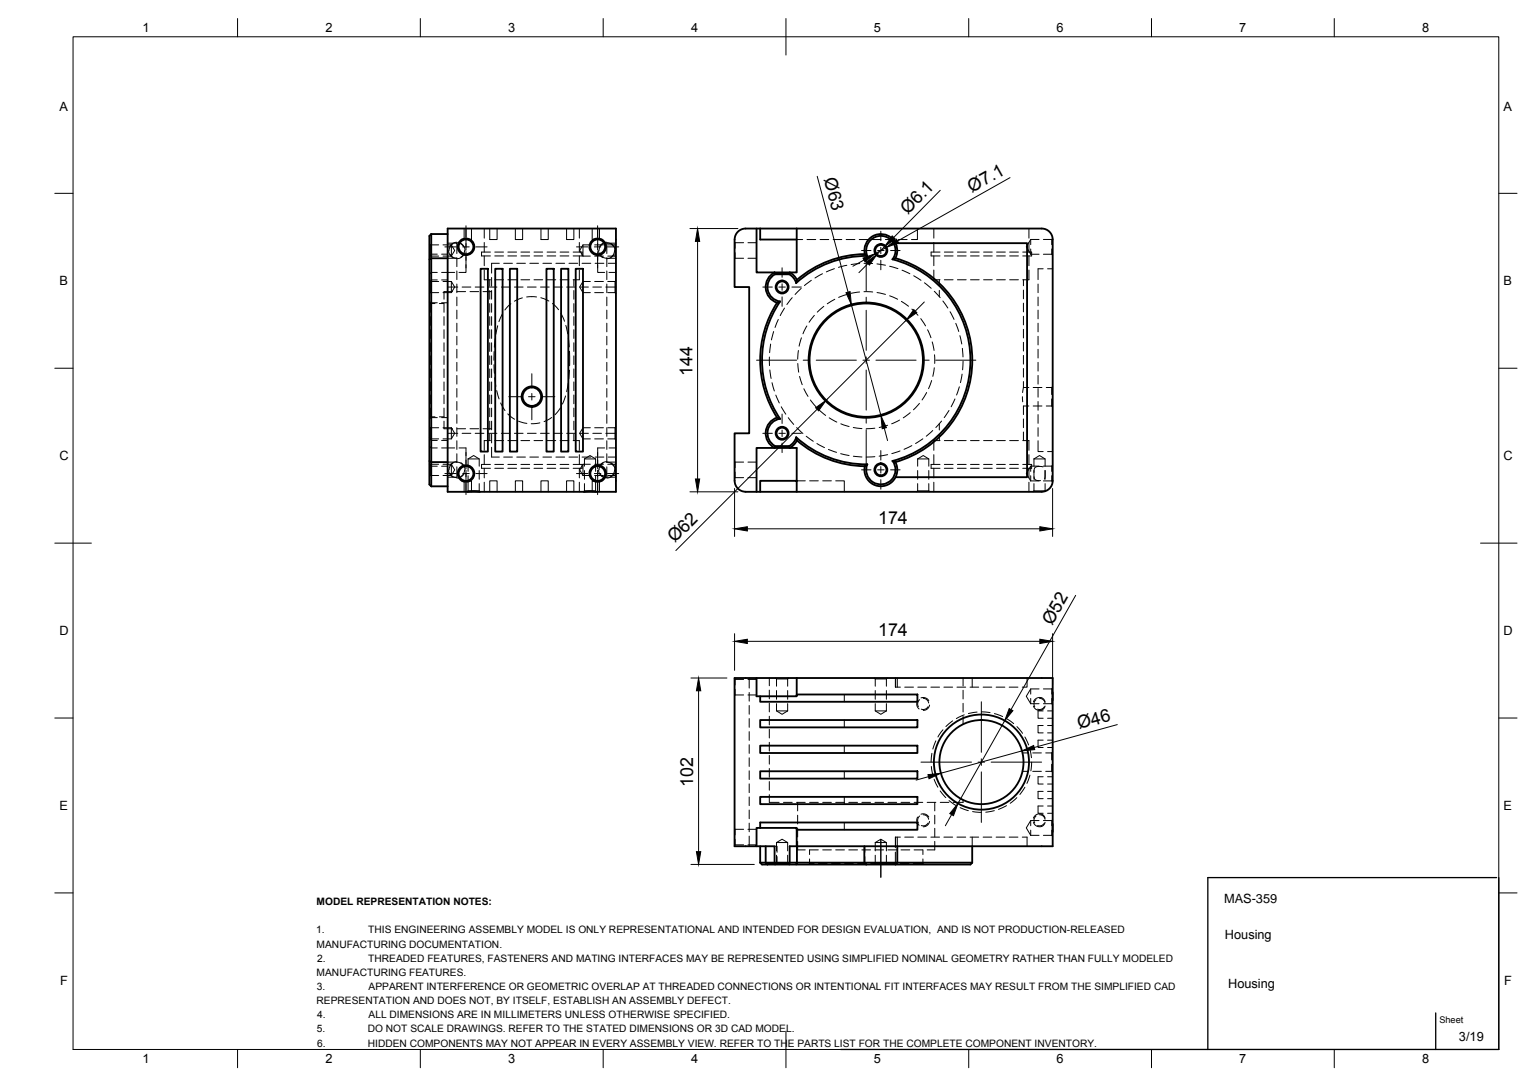
ISO-10303-21;
HEADER;
/* Generated by software containing ST-Developer
 * from STEP Tools, Inc. (www.steptools.com) 
 */

FILE_DESCRIPTION(
/* description */ (''),
/* implementation_level */ '2;1');

FILE_NAME(
/* name */ 'Housing.step',
/* time_stamp */ '2026-10-15T14:25:16-07:00',
/* author */ (''),
/* organization */ (''),
/* preprocessor_version */ 'ST-DEVELOPER v20.2',
/* originating_system */ 'Autodesk Translation Framework v15.15.0.0',
/* authorisation */ '');

FILE_SCHEMA (('AUTOMOTIVE_DESIGN { 1 0 10303 214 3 1 1 }'));
ENDSEC;

DATA;
#10=MECHANICAL_DESIGN_GEOMETRIC_PRESENTATION_REPRESENTATION('',(#323),#86429);
#287=SHAPE_REPRESENTATION_RELATIONSHIP('SRR','None',#86502,#305);
#305=ADVANCED_BREP_SHAPE_REPRESENTATION('',(#341),#86411);
#323=STYLED_ITEM('',(#86601),#341);
#341=MANIFOLD_SOLID_BREP('Body1',#15613);
#359=ELLIPSE('',#15940,151.19389506818,3.23363209990621);
#360=ELLIPSE('',#15943,151.194075359537,3.2336340714008);
#361=ELLIPSE('',#15952,151.194380471967,3.23363740533001);
#362=ELLIPSE('',#15955,151.194647853758,3.23364033017112);
#363=B_SPLINE_CURVE_WITH_KNOTS('',3,(#21563,#21564,#21565,#21566),
 .UNSPECIFIED.,.F.,.F.,(4,4),(-0.201492965018242,0.),.UNSPECIFIED.);
#364=B_SPLINE_CURVE_WITH_KNOTS('',3,(#21569,#21570,#21571,#21572),
 .UNSPECIFIED.,.F.,.F.,(4,4),(-0.195594022319034,0.),.UNSPECIFIED.);
#365=B_SPLINE_CURVE_WITH_KNOTS('',3,(#21589,#21590,#21591,#21592),
 .UNSPECIFIED.,.F.,.F.,(4,4),(-0.201492965018205,0.),.UNSPECIFIED.);
#366=B_SPLINE_CURVE_WITH_KNOTS('',3,(#21598,#21599,#21600,#21601),
 .UNSPECIFIED.,.F.,.F.,(4,4),(-0.201492965018185,0.),.UNSPECIFIED.);
#367=B_SPLINE_CURVE_WITH_KNOTS('',3,(#21620,#21621,#21622,#21623),
 .UNSPECIFIED.,.F.,.F.,(4,4),(-0.201492965018191,0.),.UNSPECIFIED.);
#368=B_SPLINE_CURVE_WITH_KNOTS('',3,(#21629,#21630,#21631,#21632),
 .UNSPECIFIED.,.F.,.F.,(4,4),(-0.195594022319061,0.),.UNSPECIFIED.);
#369=B_SPLINE_CURVE_WITH_KNOTS('',3,(#21638,#21639,#21640,#21641),
 .UNSPECIFIED.,.F.,.F.,(4,4),(-0.195594022319045,0.),.UNSPECIFIED.);
#370=B_SPLINE_CURVE_WITH_KNOTS('',3,(#21647,#21648,#21649,#21650),
 .UNSPECIFIED.,.F.,.F.,(4,4),(-0.195594022319043,0.),.UNSPECIFIED.);
#371=B_SPLINE_CURVE_WITH_KNOTS('',3,(#21681,#21682,#21683,#21684,#21685,
#21686,#21687,#21688,#21689,#21690),.UNSPECIFIED.,.F.,.F.,(4,2,2,2,4),(-3.05436467918173,
-2.86345905577985,-2.67255343237797,-2.48166347088213,-2.2907735093863),
 .UNSPECIFIED.);
#372=B_SPLINE_CURVE_WITH_KNOTS('',3,(#21691,#21692,#21693,#21694,#21695,
#21696,#21697,#21698,#21699,#21700,#21701,#21702,#21703,#21704,#21705,#21706,
#21707,#21708,#21709,#21710,#21711,#21712,#21713,#21714,#21715,#21716),
 .UNSPECIFIED.,.F.,.F.,(4,2,2,2,2,2,2,2,2,2,2,2,4),(-2.2907735093863,-2.09988354789047,
-1.90899358639463,-1.71808796299275,-1.52718233959087,-1.33627671618898,
-1.1453710927871,-0.954481131291268,-0.763591169795433,-0.572701208299599,
-0.381811246803764,-0.190905623401882,0.),.UNSPECIFIED.);
#373=B_SPLINE_CURVE_WITH_KNOTS('',3,(#21733,#21734,#21735,#21736,#21737,
#21738,#21739,#21740,#21741,#21742,#21743,#21744,#21745,#21746),
 .UNSPECIFIED.,.F.,.F.,(4,2,2,2,2,2,4),(-1.32169585665546,-1.18688181797703,
-1.0520677792986,-0.988183485413416,-0.924299191528231,-0.792573559927981,
-0.660847928327731),.UNSPECIFIED.);
#374=B_SPLINE_CURVE_WITH_KNOTS('',3,(#21748,#21749,#21750,#21751,#21752,
#21753,#21754,#21755,#21756,#21757,#21758,#21759,#21760,#21761),
 .UNSPECIFIED.,.F.,.F.,(4,2,2,2,2,2,4),(0.660847928327731,0.792573559927981,
0.924299191528231,0.988183485413416,1.0520677792986,1.18688181797703,1.32169585665546),
 .UNSPECIFIED.);
#375=B_SPLINE_CURVE_WITH_KNOTS('',3,(#21765,#21766,#21767,#21768,#21769,
#21770,#21771,#21772,#21773,#21774,#21775,#21776,#21777,#21778,#21779,#21780,
#21781,#21782,#21783,#21784,#21785,#21786,#21787,#21788,#21789,#21790,#21791),
 .UNSPECIFIED.,.F.,.F.,(4,2,2,2,2,2,3,2,2,2,2,2,4),(-0.660847928327731,
-0.529122296727481,-0.39739666512723,-0.333512371242046,-0.269628077356861,
-0.134814038678431,0.,0.13481403867843,0.269628077356861,0.333512371242045,
0.39739666512723,0.52912229672748,0.660847928327731),.UNSPECIFIED.);
#376=B_SPLINE_CURVE_WITH_KNOTS('',3,(#21798,#21799,#21800,#21801,#21802,
#21803,#21804,#21805,#21806,#21807),.UNSPECIFIED.,.F.,.F.,(4,2,2,2,4),(0.858794530961258,
0.902694826940309,1.07577532936191,1.25459835745813,1.29336839957273),
 .UNSPECIFIED.);
#377=B_SPLINE_CURVE_WITH_KNOTS('',3,(#21893,#21894,#21895,#21896,#21897,
#21898,#21899,#21900,#21901,#21902,#21903,#21904,#21905,#21906,#21907,#21908,
#21909,#21910,#21911,#21912,#21913,#21914,#21915,#21916,#21917,#21918),
 .UNSPECIFIED.,.F.,.F.,(4,2,2,2,2,2,2,2,2,2,2,2,4),(-1.32169585665546,-1.18688181797703,
-1.0520677792986,-0.988183485413416,-0.924299191528231,-0.792573559927981,
-0.660847928327731,-0.529122296727481,-0.39739666512723,-0.333512371242046,
-0.269628077356861,-0.134814038678431,0.),.UNSPECIFIED.);
#378=B_SPLINE_CURVE_WITH_KNOTS('',3,(#21919,#21920,#21921,#21922,#21923,
#21924,#21925,#21926,#21927,#21928,#21929,#21930,#21931,#21932,#21933,#21934,
#21935,#21936,#21937,#21938,#21939,#21940,#21941,#21942,#21943,#21944),
 .UNSPECIFIED.,.F.,.F.,(4,2,2,2,2,2,2,2,2,2,2,2,4),(0.,0.13481403867843,
0.269628077356861,0.333512371242045,0.39739666512723,0.52912229672748,0.660847928327731,
0.792573559927981,0.924299191528231,0.988183485413416,1.0520677792986,1.18688181797703,
1.32169585665546),.UNSPECIFIED.);
#379=B_SPLINE_CURVE_WITH_KNOTS('',3,(#21947,#21948,#21949,#21950,#21951,
#21952,#21953,#21954,#21955,#21956),.UNSPECIFIED.,.F.,.F.,(4,2,2,2,4),(0.877716942395265,
0.916486984509874,1.09531001260609,1.26839051502769,1.31229081100675),
 .UNSPECIFIED.);
#380=B_SPLINE_CURVE_WITH_KNOTS('',3,(#21958,#21959,#21960,#21961,#21962,
#21963,#21964,#21965,#21966,#21967,#21968,#21969,#21970,#21971,#21972,#21973,
#21974,#21975,#21976,#21977,#21978,#21979,#21980),.UNSPECIFIED.,.F.,.F.,
(4,2,2,2,2,3,2,2,2,2,4),(1.51638402057123,1.52276019461865,1.58643945940805,
1.65011872419746,1.7823849294906,1.91465113478373,2.04691734007687,2.17918354537001,
2.24286281015941,2.30654207494882,2.31291824899624),.UNSPECIFIED.);
#381=B_SPLINE_CURVE_WITH_KNOTS('',3,(#21981,#21982,#21983,#21984,#21985,
#21986,#21987,#21988,#21989,#21990,#21991,#21992,#21993,#21994,#21995,#21996,
#21997,#21998,#21999,#22000,#22001,#22002,#22003),.UNSPECIFIED.,.F.,.F.,
(4,2,2,2,2,3,2,2,2,2,4),(1.51638402057122,1.52276019461865,1.58643945940805,
1.65011872419746,1.7823849294906,1.91465113478373,2.04691734007687,2.17918354537001,
2.24286281015942,2.30654207494882,2.31291824899624),.UNSPECIFIED.);
#382=B_SPLINE_CURVE_WITH_KNOTS('',3,(#22016,#22017,#22018,#22019,#22020,
#22021,#22022,#22023,#22024,#22025),.UNSPECIFIED.,.F.,.F.,(4,2,2,2,4),(0.877716942395273,
0.916486984509874,1.09531001260609,1.26839051502769,1.31229081100674),
 .UNSPECIFIED.);
#383=B_SPLINE_CURVE_WITH_KNOTS('',3,(#22028,#22029,#22030,#22031,#22032,
#22033,#22034,#22035,#22036,#22037),.UNSPECIFIED.,.F.,.F.,(4,2,2,2,4),(0.858794530961249,
0.902694826940311,1.07577532936191,1.25459835745813,1.29336839957274),
 .UNSPECIFIED.);
#384=B_SPLINE_CURVE_WITH_KNOTS('',3,(#22453,#22454,#22455,#22456,#22457,
#22458,#22459,#22460,#22461,#22462,#22463,#22464,#22465,#22466,#22467,#22468,
#22469,#22470),.UNSPECIFIED.,.F.,.F.,(4,2,2,2,2,2,2,2,4),(-9.41073061373359,
-8.52189532994956,-7.63306004616553,-6.7442247623815,-5.85538947859747,
-5.5678834356648,-5.28037739273213,-4.99287134979946,-4.70536530686679),
 .UNSPECIFIED.);
#385=B_SPLINE_CURVE_WITH_KNOTS('',3,(#22472,#22473,#22474,#22475,#22476,
#22477,#22478,#22479,#22480,#22481,#22482,#22483,#22484,#22485,#22486,#22487,
#22488,#22489),.UNSPECIFIED.,.F.,.F.,(4,2,2,2,2,2,2,2,4),(4.70536530686679,
4.99287134979946,5.28037739273213,5.5678834356648,5.85538947859747,6.7442247623815,
7.63306004616553,8.52189532994956,9.41073061373359),.UNSPECIFIED.);
#386=B_SPLINE_CURVE_WITH_KNOTS('',3,(#22493,#22494,#22495,#22496,#22497,
#22498,#22499,#22500,#22501,#22502,#22503,#22504,#22505,#22506,#22507,#22508,
#22509,#22510,#22511,#22512,#22513,#22514,#22515,#22516,#22517,#22518,#22519,
#22520,#22521,#22522,#22523,#22524,#22525,#22526,#22527),.UNSPECIFIED.,
 .F.,.F.,(4,2,2,2,2,2,2,2,3,2,2,2,2,2,2,2,4),(-4.70536530686679,-4.41785926393413,
-4.13035322100146,-3.84284717806879,-3.55534113513612,-2.66650585135209,
-1.77767056756806,-0.888835283784031,0.,0.888835283784029,1.77767056756806,
2.66650585135209,3.55534113513612,3.84284717806879,4.13035322100146,4.41785926393413,
4.70536530686679),.UNSPECIFIED.);
#1145=CONICAL_SURFACE('',#15935,5.75,0.785398163397448);
#1146=CONICAL_SURFACE('',#15938,0.85,0.78539816339745);
#1147=CONICAL_SURFACE('',#15944,0.85,0.78539816339745);
#1148=CONICAL_SURFACE('',#15947,5.75,0.785398163397453);
#1149=CONICAL_SURFACE('',#15950,0.85,0.78539816339745);
#1150=CONICAL_SURFACE('',#15956,0.85,0.78539816339745);
#1151=CONICAL_SURFACE('',#15959,5.75,0.785398163397448);
#1152=CONICAL_SURFACE('',#15962,0.85,0.785398163397452);
#1153=CONICAL_SURFACE('',#15965,5.75,0.785398163397448);
#1154=CONICAL_SURFACE('',#15968,0.85,0.785398163397452);
#1155=CONICAL_SURFACE('',#15985,0.5575,0.785398163397445);
#1156=CONICAL_SURFACE('',#15987,0.2025,1.02974425867666);
#1157=CONICAL_SURFACE('',#15991,0.455,0.785398163397457);
#1158=CONICAL_SURFACE('',#16001,0.2025,1.02974425867666);
#1159=CONICAL_SURFACE('',#16005,0.455000000000001,0.785398163397459);
#1160=CONICAL_SURFACE('',#16008,0.2025,1.02974425867666);
#1161=CONICAL_SURFACE('',#16012,0.455,0.785398163397457);
#1162=CONICAL_SURFACE('',#16015,0.2025,1.02974425867666);
#1163=CONICAL_SURFACE('',#16019,0.455000000000001,0.785398163397459);
#1164=CONICAL_SURFACE('',#16020,0.1525,1.02974425867665);
#1165=CONICAL_SURFACE('',#16024,0.355,0.785398163397444);
#1166=CONICAL_SURFACE('',#16025,0.1525,1.02974425867665);
#1167=CONICAL_SURFACE('',#16029,0.355,0.785398163397446);
#1168=CONICAL_SURFACE('',#16031,0.1525,1.02974425867665);
#1169=CONICAL_SURFACE('',#16035,0.355,0.785398163397446);
#1170=CONICAL_SURFACE('',#16036,0.1525,1.02974425867665);
#1171=CONICAL_SURFACE('',#16040,0.355,0.785398163397444);
#1172=CONICAL_SURFACE('',#16042,0.1525,1.02974425867665);
#1173=CONICAL_SURFACE('',#16046,0.355,0.785398163397444);
#1174=CONICAL_SURFACE('',#16047,0.1525,1.02974425867665);
#1175=CONICAL_SURFACE('',#16051,0.355,0.785398163397444);
#1176=CONICAL_SURFACE('',#16053,0.1525,1.02974425867665);
#1177=CONICAL_SURFACE('',#16057,0.355,0.785398163397444);
#1178=CONICAL_SURFACE('',#16058,0.1525,1.02974425867665);
#1179=CONICAL_SURFACE('',#16062,0.355,0.785398163397444);
#1180=CONICAL_SURFACE('',#16064,0.1525,1.02974425867665);
#1181=CONICAL_SURFACE('',#16068,0.355,0.785398163397451);
#1182=CONICAL_SURFACE('',#16069,0.1525,1.02974425867665);
#1183=CONICAL_SURFACE('',#16073,0.355,0.785398163397448);
#1184=CONICAL_SURFACE('',#16074,0.1525,1.02974425867665);
#1185=CONICAL_SURFACE('',#16078,0.355,0.785398163397451);
#1186=CONICAL_SURFACE('',#16079,0.1525,1.02974425867665);
#1187=CONICAL_SURFACE('',#16083,0.355,0.785398163397448);
#1188=CONICAL_SURFACE('',#16087,0.462499999999999,0.785398163397447);
#1189=CONICAL_SURFACE('',#16092,0.4625,0.785398163397444);
#1190=CONICAL_SURFACE('',#16097,0.462499999999999,0.785398163397447);
#1191=CONICAL_SURFACE('',#16102,0.4625,0.785398163397444);
#1192=CONICAL_SURFACE('',#16199,3.155,0.785398163397444);
#1351=CYLINDRICAL_SURFACE('',#15906,5.8);
#1352=CYLINDRICAL_SURFACE('',#15909,0.9);
#1353=CYLINDRICAL_SURFACE('',#15915,0.9);
#1354=CYLINDRICAL_SURFACE('',#15971,0.9);
#1355=CYLINDRICAL_SURFACE('',#15972,5.8);
#1356=CYLINDRICAL_SURFACE('',#15973,0.9);
#1357=CYLINDRICAL_SURFACE('',#15974,5.8);
#1358=CYLINDRICAL_SURFACE('',#15975,0.9);
#1359=CYLINDRICAL_SURFACE('',#15976,5.8);
#1360=CYLINDRICAL_SURFACE('',#15983,0.505);
#1361=CYLINDRICAL_SURFACE('',#15989,0.405);
#1362=CYLINDRICAL_SURFACE('',#16003,0.405);
#1363=CYLINDRICAL_SURFACE('',#16006,0.6);
#1364=CYLINDRICAL_SURFACE('',#16010,0.405);
#1365=CYLINDRICAL_SURFACE('',#16013,0.6);
#1366=CYLINDRICAL_SURFACE('',#16017,0.405);
#1367=CYLINDRICAL_SURFACE('',#16022,0.305);
#1368=CYLINDRICAL_SURFACE('',#16027,0.305);
#1369=CYLINDRICAL_SURFACE('',#16033,0.305);
#1370=CYLINDRICAL_SURFACE('',#16038,0.305);
#1371=CYLINDRICAL_SURFACE('',#16044,0.305);
#1372=CYLINDRICAL_SURFACE('',#16049,0.305);
#1373=CYLINDRICAL_SURFACE('',#16055,0.305);
#1374=CYLINDRICAL_SURFACE('',#16060,0.305);
#1375=CYLINDRICAL_SURFACE('',#16066,0.305);
#1376=CYLINDRICAL_SURFACE('',#16071,0.305);
#1377=CYLINDRICAL_SURFACE('',#16076,0.305);
#1378=CYLINDRICAL_SURFACE('',#16081,0.305);
#1379=CYLINDRICAL_SURFACE('',#16084,0.425);
#1380=CYLINDRICAL_SURFACE('',#16089,0.425000000000001);
#1381=CYLINDRICAL_SURFACE('',#16094,0.425);
#1382=CYLINDRICAL_SURFACE('',#16099,0.425000000000001);
#1383=CYLINDRICAL_SURFACE('',#16120,0.9);
#1384=CYLINDRICAL_SURFACE('',#16122,0.9);
#1385=CYLINDRICAL_SURFACE('',#16123,0.9);
#1386=CYLINDRICAL_SURFACE('',#16164,2.6);
#1387=CYLINDRICAL_SURFACE('',#16168,2.75);
#1388=CYLINDRICAL_SURFACE('',#16172,2.6);
#1389=CYLINDRICAL_SURFACE('',#16176,2.3);
#1390=CYLINDRICAL_SURFACE('',#16180,2.6);
#1391=CYLINDRICAL_SURFACE('',#16184,2.75);
#1392=CYLINDRICAL_SURFACE('',#16188,2.6);
#1393=CYLINDRICAL_SURFACE('',#16189,5.3);
#1394=CYLINDRICAL_SURFACE('',#16193,3.75);
#1395=CYLINDRICAL_SURFACE('',#16197,3.1);
#1396=CYLINDRICAL_SURFACE('',#16200,5.8);
#1397=CYLINDRICAL_SURFACE('',#16201,0.6);
#1398=CYLINDRICAL_SURFACE('',#16202,0.6);
#1602=FACE_BOUND('',#3290,.T.);
#1603=FACE_BOUND('',#3291,.T.);
#1604=FACE_BOUND('',#3292,.T.);
#1605=FACE_BOUND('',#3293,.T.);
#1606=FACE_BOUND('',#3294,.T.);
#1607=FACE_BOUND('',#3328,.T.);
#1608=FACE_BOUND('',#3329,.T.);
#1609=FACE_BOUND('',#3330,.T.);
#1610=FACE_BOUND('',#3331,.T.);
#1611=FACE_BOUND('',#3332,.T.);
#1612=FACE_BOUND('',#3333,.T.);
#1613=FACE_BOUND('',#3334,.T.);
#1614=FACE_BOUND('',#3366,.T.);
#1615=FACE_BOUND('',#3367,.T.);
#1616=FACE_BOUND('',#3368,.T.);
#1617=FACE_BOUND('',#3369,.T.);
#1618=FACE_BOUND('',#3370,.T.);
#1619=FACE_BOUND('',#3377,.T.);
#1620=FACE_BOUND('',#3378,.T.);
#1621=FACE_BOUND('',#3379,.T.);
#1622=FACE_BOUND('',#3380,.T.);
#1623=FACE_BOUND('',#3381,.T.);
#1624=FACE_BOUND('',#3382,.T.);
#1625=FACE_BOUND('',#3383,.T.);
#1626=FACE_BOUND('',#3386,.T.);
#1627=FACE_BOUND('',#3428,.T.);
#1628=FACE_BOUND('',#3443,.T.);
#1629=FACE_BOUND('',#3447,.T.);
#1630=FACE_BOUND('',#3449,.T.);
#1631=FACE_BOUND('',#3450,.T.);
#1632=FACE_BOUND('',#3451,.T.);
#1633=FACE_BOUND('',#3452,.T.);
#1634=FACE_BOUND('',#3453,.T.);
#1635=FACE_BOUND('',#3454,.T.);
#1636=FACE_BOUND('',#3456,.T.);
#1637=FACE_BOUND('',#3462,.T.);
#1638=FACE_BOUND('',#3472,.T.);
#1639=FACE_BOUND('',#3473,.T.);
#1640=FACE_BOUND('',#3475,.T.);
#1641=FACE_BOUND('',#3476,.T.);
#1642=FACE_BOUND('',#3509,.T.);
#1643=FACE_BOUND('',#3512,.T.);
#1644=FACE_BOUND('',#3515,.T.);
#1645=FACE_BOUND('',#3517,.T.);
#1646=FACE_BOUND('',#3519,.T.);
#1647=FACE_BOUND('',#3522,.T.);
#1648=FACE_BOUND('',#3525,.T.);
#1649=FACE_BOUND('',#3528,.T.);
#1650=FACE_BOUND('',#3530,.T.);
#1651=FACE_BOUND('',#3533,.T.);
#1754=CIRCLE('',#15865,2.6);
#1755=CIRCLE('',#15899,0.355);
#1756=CIRCLE('',#15900,0.355);
#1757=CIRCLE('',#15901,0.355);
#1758=CIRCLE('',#15902,0.355);
#1759=CIRCLE('',#15903,2.6);
#1760=CIRCLE('',#15904,0.355);
#1761=CIRCLE('',#15905,0.355);
#1762=CIRCLE('',#15907,5.8);
#1763=CIRCLE('',#15908,5.8);
#1764=CIRCLE('',#15910,0.9);
#1765=CIRCLE('',#15911,0.9);
#1766=CIRCLE('',#15916,0.9);
#1767=CIRCLE('',#15917,0.9);
#1768=CIRCLE('',#15923,0.9);
#1769=CIRCLE('',#15924,0.9);
#1770=CIRCLE('',#15925,5.8);
#1771=CIRCLE('',#15927,0.9);
#1772=CIRCLE('',#15928,5.8);
#1773=CIRCLE('',#15929,0.9);
#1774=CIRCLE('',#15930,0.6);
#1775=CIRCLE('',#15931,0.6);
#1776=CIRCLE('',#15932,0.9);
#1777=CIRCLE('',#15933,5.8);
#1778=CIRCLE('',#15934,0.9);
#1779=CIRCLE('',#15936,5.7);
#1780=CIRCLE('',#15937,5.8);
#1781=CIRCLE('',#15939,0.8);
#1782=CIRCLE('',#15941,0.9);
#1783=CIRCLE('',#15945,0.8);
#1784=CIRCLE('',#15946,0.9);
#1785=CIRCLE('',#15948,5.7);
#1786=CIRCLE('',#15949,5.8);
#1787=CIRCLE('',#15951,0.8);
#1788=CIRCLE('',#15953,0.9);
#1789=CIRCLE('',#15957,0.9);
#1790=CIRCLE('',#15958,0.8);
#1791=CIRCLE('',#15960,5.8);
#1792=CIRCLE('',#15961,5.7);
#1793=CIRCLE('',#15963,0.9);
#1794=CIRCLE('',#15964,0.8);
#1795=CIRCLE('',#15966,5.8);
#1796=CIRCLE('',#15967,5.7);
#1797=CIRCLE('',#15969,0.9);
#1798=CIRCLE('',#15970,0.8);
#1799=CIRCLE('',#15978,3.15);
#1800=CIRCLE('',#15979,0.355);
#1801=CIRCLE('',#15980,0.355);
#1802=CIRCLE('',#15981,0.355);
#1803=CIRCLE('',#15982,0.355);
#1804=CIRCLE('',#15984,0.505);
#1805=CIRCLE('',#15986,0.559999999999998);
#1806=CIRCLE('',#15988,0.405);
#1807=CIRCLE('',#15990,0.405);
#1808=CIRCLE('',#15992,0.455);
#1809=CIRCLE('',#15993,0.455);
#1810=CIRCLE('',#15995,0.455);
#1811=CIRCLE('',#15996,0.455);
#1812=CIRCLE('',#15997,0.455000000000001);
#1813=CIRCLE('',#15998,0.455000000000001);
#1814=CIRCLE('',#15999,0.455000000000001);
#1815=CIRCLE('',#16000,0.455000000000001);
#1816=CIRCLE('',#16002,0.405);
#1817=CIRCLE('',#16004,0.405);
#1818=CIRCLE('',#16007,0.6);
#1819=CIRCLE('',#16009,0.405);
#1820=CIRCLE('',#16011,0.405);
#1821=CIRCLE('',#16014,0.6);
#1822=CIRCLE('',#16016,0.405);
#1823=CIRCLE('',#16018,0.405);
#1824=CIRCLE('',#16021,0.305);
#1825=CIRCLE('',#16023,0.305);
#1826=CIRCLE('',#16026,0.305);
#1827=CIRCLE('',#16028,0.305);
#1828=CIRCLE('',#16030,0.355);
#1829=CIRCLE('',#16032,0.305);
#1830=CIRCLE('',#16034,0.305);
#1831=CIRCLE('',#16037,0.305);
#1832=CIRCLE('',#16039,0.305);
#1833=CIRCLE('',#16041,0.355);
#1834=CIRCLE('',#16043,0.305);
#1835=CIRCLE('',#16045,0.305);
#1836=CIRCLE('',#16048,0.305);
#1837=CIRCLE('',#16050,0.305);
#1838=CIRCLE('',#16052,0.355);
#1839=CIRCLE('',#16054,0.305);
#1840=CIRCLE('',#16056,0.305);
#1841=CIRCLE('',#16059,0.305);
#1842=CIRCLE('',#16061,0.305);
#1843=CIRCLE('',#16063,0.355);
#1844=CIRCLE('',#16065,0.305);
#1845=CIRCLE('',#16067,0.305);
#1846=CIRCLE('',#16070,0.305);
#1847=CIRCLE('',#16072,0.305);
#1848=CIRCLE('',#16075,0.305);
#1849=CIRCLE('',#16077,0.305);
#1850=CIRCLE('',#16080,0.305);
#1851=CIRCLE('',#16082,0.305);
#1852=CIRCLE('',#16085,0.425);
#1853=CIRCLE('',#16086,0.425);
#1854=CIRCLE('',#16088,0.45);
#1855=CIRCLE('',#16090,0.425000000000001);
#1856=CIRCLE('',#16091,0.425000000000001);
#1857=CIRCLE('',#16093,0.45);
#1858=CIRCLE('',#16095,0.425);
#1859=CIRCLE('',#16096,0.425);
#1860=CIRCLE('',#16098,0.45);
#1861=CIRCLE('',#16100,0.425000000000001);
#1862=CIRCLE('',#16101,0.425000000000001);
#1863=CIRCLE('',#16103,0.45);
#1864=CIRCLE('',#16110,0.6);
#1865=CIRCLE('',#16111,0.6);
#1866=CIRCLE('',#16112,5.3);
#1867=CIRCLE('',#16121,0.9);
#1868=CIRCLE('',#16124,0.9);
#1869=CIRCLE('',#16126,0.6);
#1870=CIRCLE('',#16127,0.6);
#1871=CIRCLE('',#16128,5.8);
#1872=CIRCLE('',#16165,2.6);
#1873=CIRCLE('',#16167,2.75);
#1874=CIRCLE('',#16169,2.75);
#1875=CIRCLE('',#16171,2.6);
#1876=CIRCLE('',#16173,2.6);
#1877=CIRCLE('',#16175,2.3);
#1878=CIRCLE('',#16177,2.3);
#1879=CIRCLE('',#16179,2.6);
#1880=CIRCLE('',#16181,2.6);
#1881=CIRCLE('',#16183,2.75);
#1882=CIRCLE('',#16185,2.75);
#1883=CIRCLE('',#16187,2.6);
#1884=CIRCLE('',#16190,5.3);
#1885=CIRCLE('',#16192,3.75);
#1886=CIRCLE('',#16194,3.75);
#1887=CIRCLE('',#16196,3.1);
#1888=CIRCLE('',#16198,3.1);
#2385=FACE_OUTER_BOUND('',#3257,.T.);
#2386=FACE_OUTER_BOUND('',#3258,.T.);
#2387=FACE_OUTER_BOUND('',#3259,.T.);
#2388=FACE_OUTER_BOUND('',#3260,.T.);
#2389=FACE_OUTER_BOUND('',#3261,.T.);
#2390=FACE_OUTER_BOUND('',#3262,.T.);
#2391=FACE_OUTER_BOUND('',#3263,.T.);
#2392=FACE_OUTER_BOUND('',#3264,.T.);
#2393=FACE_OUTER_BOUND('',#3265,.T.);
#2394=FACE_OUTER_BOUND('',#3266,.T.);
#2395=FACE_OUTER_BOUND('',#3267,.T.);
#2396=FACE_OUTER_BOUND('',#3268,.T.);
#2397=FACE_OUTER_BOUND('',#3269,.T.);
#2398=FACE_OUTER_BOUND('',#3270,.T.);
#2399=FACE_OUTER_BOUND('',#3271,.T.);
#2400=FACE_OUTER_BOUND('',#3272,.T.);
#2401=FACE_OUTER_BOUND('',#3273,.T.);
#2402=FACE_OUTER_BOUND('',#3274,.T.);
#2403=FACE_OUTER_BOUND('',#3275,.T.);
#2404=FACE_OUTER_BOUND('',#3276,.T.);
#2405=FACE_OUTER_BOUND('',#3277,.T.);
#2406=FACE_OUTER_BOUND('',#3278,.T.);
#2407=FACE_OUTER_BOUND('',#3279,.T.);
#2408=FACE_OUTER_BOUND('',#3280,.T.);
#2409=FACE_OUTER_BOUND('',#3281,.T.);
#2410=FACE_OUTER_BOUND('',#3282,.T.);
#2411=FACE_OUTER_BOUND('',#3283,.T.);
#2412=FACE_OUTER_BOUND('',#3284,.T.);
#2413=FACE_OUTER_BOUND('',#3285,.T.);
#2414=FACE_OUTER_BOUND('',#3286,.T.);
#2415=FACE_OUTER_BOUND('',#3287,.T.);
#2416=FACE_OUTER_BOUND('',#3288,.T.);
#2417=FACE_OUTER_BOUND('',#3289,.T.);
#2418=FACE_OUTER_BOUND('',#3295,.T.);
#2419=FACE_OUTER_BOUND('',#3296,.T.);
#2420=FACE_OUTER_BOUND('',#3297,.T.);
#2421=FACE_OUTER_BOUND('',#3298,.T.);
#2422=FACE_OUTER_BOUND('',#3299,.T.);
#2423=FACE_OUTER_BOUND('',#3300,.T.);
#2424=FACE_OUTER_BOUND('',#3301,.T.);
#2425=FACE_OUTER_BOUND('',#3302,.T.);
#2426=FACE_OUTER_BOUND('',#3303,.T.);
#2427=FACE_OUTER_BOUND('',#3304,.T.);
#2428=FACE_OUTER_BOUND('',#3305,.T.);
#2429=FACE_OUTER_BOUND('',#3306,.T.);
#2430=FACE_OUTER_BOUND('',#3307,.T.);
#2431=FACE_OUTER_BOUND('',#3308,.T.);
#2432=FACE_OUTER_BOUND('',#3309,.T.);
#2433=FACE_OUTER_BOUND('',#3310,.T.);
#2434=FACE_OUTER_BOUND('',#3311,.T.);
#2435=FACE_OUTER_BOUND('',#3312,.T.);
#2436=FACE_OUTER_BOUND('',#3313,.T.);
#2437=FACE_OUTER_BOUND('',#3314,.T.);
#2438=FACE_OUTER_BOUND('',#3315,.T.);
#2439=FACE_OUTER_BOUND('',#3316,.T.);
#2440=FACE_OUTER_BOUND('',#3317,.T.);
#2441=FACE_OUTER_BOUND('',#3318,.T.);
#2442=FACE_OUTER_BOUND('',#3319,.T.);
#2443=FACE_OUTER_BOUND('',#3320,.T.);
#2444=FACE_OUTER_BOUND('',#3321,.T.);
#2445=FACE_OUTER_BOUND('',#3322,.T.);
#2446=FACE_OUTER_BOUND('',#3323,.T.);
#2447=FACE_OUTER_BOUND('',#3324,.T.);
#2448=FACE_OUTER_BOUND('',#3325,.T.);
#2449=FACE_OUTER_BOUND('',#3326,.T.);
#2450=FACE_OUTER_BOUND('',#3327,.T.);
#2451=FACE_OUTER_BOUND('',#3335,.T.);
#2452=FACE_OUTER_BOUND('',#3336,.T.);
#2453=FACE_OUTER_BOUND('',#3337,.T.);
#2454=FACE_OUTER_BOUND('',#3338,.T.);
#2455=FACE_OUTER_BOUND('',#3339,.T.);
#2456=FACE_OUTER_BOUND('',#3340,.T.);
#2457=FACE_OUTER_BOUND('',#3341,.T.);
#2458=FACE_OUTER_BOUND('',#3342,.T.);
#2459=FACE_OUTER_BOUND('',#3343,.T.);
#2460=FACE_OUTER_BOUND('',#3344,.T.);
#2461=FACE_OUTER_BOUND('',#3345,.T.);
#2462=FACE_OUTER_BOUND('',#3346,.T.);
#2463=FACE_OUTER_BOUND('',#3347,.T.);
#2464=FACE_OUTER_BOUND('',#3348,.T.);
#2465=FACE_OUTER_BOUND('',#3349,.T.);
#2466=FACE_OUTER_BOUND('',#3350,.T.);
#2467=FACE_OUTER_BOUND('',#3351,.T.);
#2468=FACE_OUTER_BOUND('',#3352,.T.);
#2469=FACE_OUTER_BOUND('',#3353,.T.);
#2470=FACE_OUTER_BOUND('',#3354,.T.);
#2471=FACE_OUTER_BOUND('',#3355,.T.);
#2472=FACE_OUTER_BOUND('',#3356,.T.);
#2473=FACE_OUTER_BOUND('',#3357,.T.);
#2474=FACE_OUTER_BOUND('',#3358,.T.);
#2475=FACE_OUTER_BOUND('',#3359,.T.);
#2476=FACE_OUTER_BOUND('',#3360,.T.);
#2477=FACE_OUTER_BOUND('',#3361,.T.);
#2478=FACE_OUTER_BOUND('',#3362,.T.);
#2479=FACE_OUTER_BOUND('',#3363,.T.);
#2480=FACE_OUTER_BOUND('',#3364,.T.);
#2481=FACE_OUTER_BOUND('',#3365,.T.);
#2482=FACE_OUTER_BOUND('',#3371,.T.);
#2483=FACE_OUTER_BOUND('',#3372,.T.);
#2484=FACE_OUTER_BOUND('',#3373,.T.);
#2485=FACE_OUTER_BOUND('',#3374,.T.);
#2486=FACE_OUTER_BOUND('',#3375,.T.);
#2487=FACE_OUTER_BOUND('',#3376,.T.);
#2488=FACE_OUTER_BOUND('',#3384,.T.);
#2489=FACE_OUTER_BOUND('',#3385,.T.);
#2490=FACE_OUTER_BOUND('',#3387,.T.);
#2491=FACE_OUTER_BOUND('',#3388,.T.);
#2492=FACE_OUTER_BOUND('',#3389,.T.);
#2493=FACE_OUTER_BOUND('',#3390,.T.);
#2494=FACE_OUTER_BOUND('',#3391,.T.);
#2495=FACE_OUTER_BOUND('',#3392,.T.);
#2496=FACE_OUTER_BOUND('',#3393,.T.);
#2497=FACE_OUTER_BOUND('',#3394,.T.);
#2498=FACE_OUTER_BOUND('',#3395,.T.);
#2499=FACE_OUTER_BOUND('',#3396,.T.);
#2500=FACE_OUTER_BOUND('',#3397,.T.);
#2501=FACE_OUTER_BOUND('',#3398,.T.);
#2502=FACE_OUTER_BOUND('',#3399,.T.);
#2503=FACE_OUTER_BOUND('',#3400,.T.);
#2504=FACE_OUTER_BOUND('',#3401,.T.);
#2505=FACE_OUTER_BOUND('',#3402,.T.);
#2506=FACE_OUTER_BOUND('',#3403,.T.);
#2507=FACE_OUTER_BOUND('',#3404,.T.);
#2508=FACE_OUTER_BOUND('',#3405,.T.);
#2509=FACE_OUTER_BOUND('',#3406,.T.);
#2510=FACE_OUTER_BOUND('',#3407,.T.);
#2511=FACE_OUTER_BOUND('',#3408,.T.);
#2512=FACE_OUTER_BOUND('',#3409,.T.);
#2513=FACE_OUTER_BOUND('',#3410,.T.);
#2514=FACE_OUTER_BOUND('',#3411,.T.);
#2515=FACE_OUTER_BOUND('',#3412,.T.);
#2516=FACE_OUTER_BOUND('',#3413,.T.);
#2517=FACE_OUTER_BOUND('',#3414,.T.);
#2518=FACE_OUTER_BOUND('',#3415,.T.);
#2519=FACE_OUTER_BOUND('',#3416,.T.);
#2520=FACE_OUTER_BOUND('',#3417,.T.);
#2521=FACE_OUTER_BOUND('',#3418,.T.);
#2522=FACE_OUTER_BOUND('',#3419,.T.);
#2523=FACE_OUTER_BOUND('',#3420,.T.);
#2524=FACE_OUTER_BOUND('',#3421,.T.);
#2525=FACE_OUTER_BOUND('',#3422,.T.);
#2526=FACE_OUTER_BOUND('',#3423,.T.);
#2527=FACE_OUTER_BOUND('',#3424,.T.);
#2528=FACE_OUTER_BOUND('',#3425,.T.);
#2529=FACE_OUTER_BOUND('',#3426,.T.);
#2530=FACE_OUTER_BOUND('',#3427,.T.);
#2531=FACE_OUTER_BOUND('',#3429,.T.);
#2532=FACE_OUTER_BOUND('',#3430,.T.);
#2533=FACE_OUTER_BOUND('',#3431,.T.);
#2534=FACE_OUTER_BOUND('',#3432,.T.);
#2535=FACE_OUTER_BOUND('',#3433,.T.);
#2536=FACE_OUTER_BOUND('',#3434,.T.);
#2537=FACE_OUTER_BOUND('',#3435,.T.);
#2538=FACE_OUTER_BOUND('',#3436,.T.);
#2539=FACE_OUTER_BOUND('',#3437,.T.);
#2540=FACE_OUTER_BOUND('',#3438,.T.);
#2541=FACE_OUTER_BOUND('',#3439,.T.);
#2542=FACE_OUTER_BOUND('',#3440,.T.);
#2543=FACE_OUTER_BOUND('',#3441,.T.);
#2544=FACE_OUTER_BOUND('',#3442,.T.);
#2545=FACE_OUTER_BOUND('',#3444,.T.);
#2546=FACE_OUTER_BOUND('',#3445,.T.);
#2547=FACE_OUTER_BOUND('',#3446,.T.);
#2548=FACE_OUTER_BOUND('',#3448,.T.);
#2549=FACE_OUTER_BOUND('',#3455,.T.);
#2550=FACE_OUTER_BOUND('',#3457,.T.);
#2551=FACE_OUTER_BOUND('',#3458,.T.);
#2552=FACE_OUTER_BOUND('',#3459,.T.);
#2553=FACE_OUTER_BOUND('',#3460,.T.);
#2554=FACE_OUTER_BOUND('',#3461,.T.);
#2555=FACE_OUTER_BOUND('',#3463,.T.);
#2556=FACE_OUTER_BOUND('',#3464,.T.);
#2557=FACE_OUTER_BOUND('',#3465,.T.);
#2558=FACE_OUTER_BOUND('',#3466,.T.);
#2559=FACE_OUTER_BOUND('',#3467,.T.);
#2560=FACE_OUTER_BOUND('',#3468,.T.);
#2561=FACE_OUTER_BOUND('',#3469,.T.);
#2562=FACE_OUTER_BOUND('',#3470,.T.);
#2563=FACE_OUTER_BOUND('',#3471,.T.);
#2564=FACE_OUTER_BOUND('',#3474,.T.);
#2565=FACE_OUTER_BOUND('',#3477,.T.);
#2566=FACE_OUTER_BOUND('',#3478,.T.);
#2567=FACE_OUTER_BOUND('',#3479,.T.);
#2568=FACE_OUTER_BOUND('',#3480,.T.);
#2569=FACE_OUTER_BOUND('',#3481,.T.);
#2570=FACE_OUTER_BOUND('',#3482,.T.);
#2571=FACE_OUTER_BOUND('',#3483,.T.);
#2572=FACE_OUTER_BOUND('',#3484,.T.);
#2573=FACE_OUTER_BOUND('',#3485,.T.);
#2574=FACE_OUTER_BOUND('',#3486,.T.);
#2575=FACE_OUTER_BOUND('',#3487,.T.);
#2576=FACE_OUTER_BOUND('',#3488,.T.);
#2577=FACE_OUTER_BOUND('',#3489,.T.);
#2578=FACE_OUTER_BOUND('',#3490,.T.);
#2579=FACE_OUTER_BOUND('',#3491,.T.);
#2580=FACE_OUTER_BOUND('',#3492,.T.);
#2581=FACE_OUTER_BOUND('',#3493,.T.);
#2582=FACE_OUTER_BOUND('',#3494,.T.);
#2583=FACE_OUTER_BOUND('',#3495,.T.);
#2584=FACE_OUTER_BOUND('',#3496,.T.);
#2585=FACE_OUTER_BOUND('',#3497,.T.);
#2586=FACE_OUTER_BOUND('',#3498,.T.);
#2587=FACE_OUTER_BOUND('',#3499,.T.);
#2588=FACE_OUTER_BOUND('',#3500,.T.);
#2589=FACE_OUTER_BOUND('',#3501,.T.);
#2590=FACE_OUTER_BOUND('',#3502,.T.);
#2591=FACE_OUTER_BOUND('',#3503,.T.);
#2592=FACE_OUTER_BOUND('',#3504,.T.);
#2593=FACE_OUTER_BOUND('',#3505,.T.);
#2594=FACE_OUTER_BOUND('',#3506,.T.);
#2595=FACE_OUTER_BOUND('',#3507,.T.);
#2596=FACE_OUTER_BOUND('',#3508,.T.);
#2597=FACE_OUTER_BOUND('',#3510,.T.);
#2598=FACE_OUTER_BOUND('',#3511,.T.);
#2599=FACE_OUTER_BOUND('',#3513,.T.);
#2600=FACE_OUTER_BOUND('',#3514,.T.);
#2601=FACE_OUTER_BOUND('',#3516,.T.);
#2602=FACE_OUTER_BOUND('',#3518,.T.);
#2603=FACE_OUTER_BOUND('',#3520,.T.);
#2604=FACE_OUTER_BOUND('',#3521,.T.);
#2605=FACE_OUTER_BOUND('',#3523,.T.);
#2606=FACE_OUTER_BOUND('',#3524,.T.);
#2607=FACE_OUTER_BOUND('',#3526,.T.);
#2608=FACE_OUTER_BOUND('',#3527,.T.);
#2609=FACE_OUTER_BOUND('',#3529,.T.);
#2610=FACE_OUTER_BOUND('',#3531,.T.);
#2611=FACE_OUTER_BOUND('',#3532,.T.);
#2612=FACE_OUTER_BOUND('',#3534,.T.);
#2613=FACE_OUTER_BOUND('',#3535,.T.);
#2614=FACE_OUTER_BOUND('',#3536,.T.);
#2615=FACE_OUTER_BOUND('',#3537,.T.);
#2616=FACE_OUTER_BOUND('',#3538,.T.);
#3257=EDGE_LOOP('',(#9851,#9852,#9853,#9854));
#3258=EDGE_LOOP('',(#9855,#9856,#9857,#9858));
#3259=EDGE_LOOP('',(#9859,#9860,#9861,#9862));
#3260=EDGE_LOOP('',(#9863,#9864,#9865,#9866));
#3261=EDGE_LOOP('',(#9867,#9868,#9869,#9870));
#3262=EDGE_LOOP('',(#9871,#9872,#9873,#9874));
#3263=EDGE_LOOP('',(#9875,#9876,#9877,#9878,#9879,#9880));
#3264=EDGE_LOOP('',(#9881,#9882,#9883,#9884));
#3265=EDGE_LOOP('',(#9885,#9886,#9887,#9888));
#3266=EDGE_LOOP('',(#9889,#9890,#9891,#9892));
#3267=EDGE_LOOP('',(#9893,#9894,#9895,#9896));
#3268=EDGE_LOOP('',(#9897,#9898,#9899,#9900));
#3269=EDGE_LOOP('',(#9901,#9902,#9903,#9904));
#3270=EDGE_LOOP('',(#9905,#9906,#9907,#9908));
#3271=EDGE_LOOP('',(#9909,#9910,#9911,#9912));
#3272=EDGE_LOOP('',(#9913,#9914,#9915,#9916));
#3273=EDGE_LOOP('',(#9917,#9918,#9919,#9920));
#3274=EDGE_LOOP('',(#9921,#9922,#9923,#9924));
#3275=EDGE_LOOP('',(#9925,#9926,#9927,#9928));
#3276=EDGE_LOOP('',(#9929,#9930,#9931,#9932));
#3277=EDGE_LOOP('',(#9933,#9934,#9935,#9936));
#3278=EDGE_LOOP('',(#9937,#9938,#9939,#9940));
#3279=EDGE_LOOP('',(#9941,#9942,#9943,#9944));
#3280=EDGE_LOOP('',(#9945,#9946,#9947,#9948));
#3281=EDGE_LOOP('',(#9949,#9950,#9951,#9952));
#3282=EDGE_LOOP('',(#9953,#9954,#9955,#9956));
#3283=EDGE_LOOP('',(#9957,#9958,#9959,#9960));
#3284=EDGE_LOOP('',(#9961,#9962,#9963,#9964));
#3285=EDGE_LOOP('',(#9965,#9966,#9967,#9968));
#3286=EDGE_LOOP('',(#9969,#9970,#9971,#9972,#9973,#9974));
#3287=EDGE_LOOP('',(#9975,#9976,#9977,#9978,#9979,#9980));
#3288=EDGE_LOOP('',(#9981,#9982,#9983,#9984,#9985,#9986));
#3289=EDGE_LOOP('',(#9987,#9988,#9989,#9990,#9991,#9992,#9993,#9994,#9995,
#9996,#9997,#9998,#9999,#10000,#10001,#10002,#10003,#10004,#10005,#10006));
#3290=EDGE_LOOP('',(#10007));
#3291=EDGE_LOOP('',(#10008,#10009,#10010,#10011));
#3292=EDGE_LOOP('',(#10012,#10013,#10014,#10015));
#3293=EDGE_LOOP('',(#10016,#10017,#10018,#10019));
#3294=EDGE_LOOP('',(#10020,#10021,#10022,#10023));
#3295=EDGE_LOOP('',(#10024,#10025,#10026,#10027));
#3296=EDGE_LOOP('',(#10028,#10029,#10030,#10031));
#3297=EDGE_LOOP('',(#10032,#10033,#10034,#10035));
#3298=EDGE_LOOP('',(#10036,#10037,#10038,#10039));
#3299=EDGE_LOOP('',(#10040,#10041,#10042,#10043));
#3300=EDGE_LOOP('',(#10044,#10045,#10046,#10047));
#3301=EDGE_LOOP('',(#10048,#10049,#10050,#10051));
#3302=EDGE_LOOP('',(#10052,#10053,#10054,#10055));
#3303=EDGE_LOOP('',(#10056,#10057,#10058,#10059));
#3304=EDGE_LOOP('',(#10060,#10061,#10062,#10063,#10064,#10065));
#3305=EDGE_LOOP('',(#10066,#10067,#10068,#10069));
#3306=EDGE_LOOP('',(#10070,#10071,#10072,#10073));
#3307=EDGE_LOOP('',(#10074,#10075,#10076,#10077));
#3308=EDGE_LOOP('',(#10078,#10079,#10080,#10081));
#3309=EDGE_LOOP('',(#10082,#10083,#10084,#10085));
#3310=EDGE_LOOP('',(#10086,#10087,#10088,#10089));
#3311=EDGE_LOOP('',(#10090,#10091,#10092,#10093));
#3312=EDGE_LOOP('',(#10094,#10095,#10096,#10097));
#3313=EDGE_LOOP('',(#10098,#10099,#10100,#10101));
#3314=EDGE_LOOP('',(#10102,#10103,#10104,#10105));
#3315=EDGE_LOOP('',(#10106,#10107,#10108,#10109));
#3316=EDGE_LOOP('',(#10110,#10111,#10112,#10113));
#3317=EDGE_LOOP('',(#10114,#10115,#10116,#10117));
#3318=EDGE_LOOP('',(#10118,#10119,#10120,#10121));
#3319=EDGE_LOOP('',(#10122,#10123,#10124,#10125));
#3320=EDGE_LOOP('',(#10126,#10127,#10128,#10129));
#3321=EDGE_LOOP('',(#10130,#10131,#10132,#10133));
#3322=EDGE_LOOP('',(#10134,#10135,#10136,#10137));
#3323=EDGE_LOOP('',(#10138,#10139,#10140,#10141));
#3324=EDGE_LOOP('',(#10142,#10143,#10144,#10145,#10146,#10147));
#3325=EDGE_LOOP('',(#10148,#10149,#10150,#10151,#10152,#10153));
#3326=EDGE_LOOP('',(#10154,#10155,#10156,#10157,#10158,#10159));
#3327=EDGE_LOOP('',(#10160,#10161,#10162,#10163,#10164,#10165,#10166,#10167,
#10168,#10169,#10170,#10171,#10172,#10173,#10174,#10175,#10176,#10177,#10178,
#10179,#10180,#10181,#10182,#10183,#10184,#10185));
#3328=EDGE_LOOP('',(#10186));
#3329=EDGE_LOOP('',(#10187));
#3330=EDGE_LOOP('',(#10188));
#3331=EDGE_LOOP('',(#10189,#10190,#10191,#10192));
#3332=EDGE_LOOP('',(#10193,#10194,#10195,#10196));
#3333=EDGE_LOOP('',(#10197,#10198,#10199,#10200));
#3334=EDGE_LOOP('',(#10201,#10202,#10203,#10204));
#3335=EDGE_LOOP('',(#10205,#10206,#10207,#10208));
#3336=EDGE_LOOP('',(#10209,#10210,#10211,#10212));
#3337=EDGE_LOOP('',(#10213,#10214,#10215,#10216));
#3338=EDGE_LOOP('',(#10217,#10218,#10219,#10220));
#3339=EDGE_LOOP('',(#10221,#10222,#10223,#10224));
#3340=EDGE_LOOP('',(#10225,#10226,#10227,#10228));
#3341=EDGE_LOOP('',(#10229,#10230,#10231,#10232,#10233,#10234));
#3342=EDGE_LOOP('',(#10235,#10236,#10237,#10238));
#3343=EDGE_LOOP('',(#10239,#10240,#10241,#10242));
#3344=EDGE_LOOP('',(#10243,#10244,#10245,#10246));
#3345=EDGE_LOOP('',(#10247,#10248,#10249,#10250,#10251,#10252));
#3346=EDGE_LOOP('',(#10253,#10254,#10255,#10256,#10257,#10258,#10259,#10260,
#10261,#10262,#10263,#10264,#10265,#10266,#10267,#10268,#10269,#10270));
#3347=EDGE_LOOP('',(#10271,#10272,#10273,#10274));
#3348=EDGE_LOOP('',(#10275,#10276,#10277,#10278));
#3349=EDGE_LOOP('',(#10279,#10280,#10281,#10282));
#3350=EDGE_LOOP('',(#10283,#10284,#10285,#10286));
#3351=EDGE_LOOP('',(#10287,#10288,#10289,#10290));
#3352=EDGE_LOOP('',(#10291,#10292,#10293,#10294));
#3353=EDGE_LOOP('',(#10295,#10296,#10297,#10298));
#3354=EDGE_LOOP('',(#10299,#10300,#10301,#10302));
#3355=EDGE_LOOP('',(#10303,#10304,#10305,#10306));
#3356=EDGE_LOOP('',(#10307,#10308,#10309,#10310));
#3357=EDGE_LOOP('',(#10311,#10312,#10313,#10314));
#3358=EDGE_LOOP('',(#10315,#10316,#10317,#10318));
#3359=EDGE_LOOP('',(#10319,#10320,#10321,#10322));
#3360=EDGE_LOOP('',(#10323,#10324,#10325,#10326));
#3361=EDGE_LOOP('',(#10327,#10328,#10329,#10330,#10331,#10332));
#3362=EDGE_LOOP('',(#10333,#10334,#10335,#10336));
#3363=EDGE_LOOP('',(#10337,#10338,#10339,#10340,#10341,#10342));
#3364=EDGE_LOOP('',(#10343,#10344,#10345,#10346));
#3365=EDGE_LOOP('',(#10347,#10348,#10349,#10350,#10351,#10352,#10353,#10354,
#10355,#10356,#10357,#10358));
#3366=EDGE_LOOP('',(#10359));
#3367=EDGE_LOOP('',(#10360));
#3368=EDGE_LOOP('',(#10361));
#3369=EDGE_LOOP('',(#10362));
#3370=EDGE_LOOP('',(#10363));
#3371=EDGE_LOOP('',(#10364,#10365,#10366,#10367,#10368));
#3372=EDGE_LOOP('',(#10369,#10370,#10371,#10372));
#3373=EDGE_LOOP('',(#10373,#10374,#10375));
#3374=EDGE_LOOP('',(#10376,#10377,#10378,#10379,#10380,#10381,#10382,#10383,
#10384));
#3375=EDGE_LOOP('',(#10385,#10386,#10387,#10388,#10389,#10390));
#3376=EDGE_LOOP('',(#10391,#10392,#10393,#10394,#10395,#10396,#10397,#10398,
#10399,#10400,#10401,#10402,#10403,#10404,#10405,#10406));
#3377=EDGE_LOOP('',(#10407));
#3378=EDGE_LOOP('',(#10408,#10409,#10410,#10411));
#3379=EDGE_LOOP('',(#10412,#10413,#10414,#10415));
#3380=EDGE_LOOP('',(#10416,#10417,#10418,#10419));
#3381=EDGE_LOOP('',(#10420,#10421,#10422,#10423));
#3382=EDGE_LOOP('',(#10424,#10425,#10426,#10427));
#3383=EDGE_LOOP('',(#10428,#10429,#10430,#10431));
#3384=EDGE_LOOP('',(#10432,#10433,#10434));
#3385=EDGE_LOOP('',(#10435,#10436,#10437,#10438));
#3386=EDGE_LOOP('',(#10439,#10440));
#3387=EDGE_LOOP('',(#10441,#10442,#10443,#10444,#10445,#10446));
#3388=EDGE_LOOP('',(#10447,#10448,#10449,#10450,#10451,#10452,#10453,#10454,
#10455,#10456,#10457,#10458));
#3389=EDGE_LOOP('',(#10459,#10460,#10461));
#3390=EDGE_LOOP('',(#10462,#10463,#10464,#10465));
#3391=EDGE_LOOP('',(#10466,#10467,#10468,#10469,#10470,#10471));
#3392=EDGE_LOOP('',(#10472,#10473,#10474,#10475,#10476,#10477,#10478,#10479));
#3393=EDGE_LOOP('',(#10480,#10481,#10482));
#3394=EDGE_LOOP('',(#10483,#10484,#10485,#10486));
#3395=EDGE_LOOP('',(#10487,#10488,#10489,#10490,#10491,#10492));
#3396=EDGE_LOOP('',(#10493,#10494,#10495));
#3397=EDGE_LOOP('',(#10496,#10497,#10498,#10499));
#3398=EDGE_LOOP('',(#10500,#10501,#10502,#10503));
#3399=EDGE_LOOP('',(#10504,#10505,#10506));
#3400=EDGE_LOOP('',(#10507,#10508,#10509,#10510));
#3401=EDGE_LOOP('',(#10511,#10512,#10513,#10514));
#3402=EDGE_LOOP('',(#10515,#10516,#10517));
#3403=EDGE_LOOP('',(#10518,#10519,#10520,#10521));
#3404=EDGE_LOOP('',(#10522,#10523,#10524,#10525));
#3405=EDGE_LOOP('',(#10526,#10527,#10528));
#3406=EDGE_LOOP('',(#10529,#10530,#10531,#10532));
#3407=EDGE_LOOP('',(#10533,#10534,#10535,#10536));
#3408=EDGE_LOOP('',(#10537,#10538,#10539));
#3409=EDGE_LOOP('',(#10540,#10541,#10542,#10543));
#3410=EDGE_LOOP('',(#10544,#10545,#10546,#10547));
#3411=EDGE_LOOP('',(#10548,#10549,#10550));
#3412=EDGE_LOOP('',(#10551,#10552,#10553,#10554));
#3413=EDGE_LOOP('',(#10555,#10556,#10557,#10558));
#3414=EDGE_LOOP('',(#10559,#10560,#10561));
#3415=EDGE_LOOP('',(#10562,#10563,#10564,#10565));
#3416=EDGE_LOOP('',(#10566,#10567,#10568,#10569));
#3417=EDGE_LOOP('',(#10570,#10571,#10572));
#3418=EDGE_LOOP('',(#10573,#10574,#10575,#10576));
#3419=EDGE_LOOP('',(#10577,#10578,#10579,#10580));
#3420=EDGE_LOOP('',(#10581,#10582,#10583));
#3421=EDGE_LOOP('',(#10584,#10585,#10586,#10587));
#3422=EDGE_LOOP('',(#10588,#10589,#10590,#10591));
#3423=EDGE_LOOP('',(#10592,#10593,#10594));
#3424=EDGE_LOOP('',(#10595,#10596,#10597,#10598));
#3425=EDGE_LOOP('',(#10599,#10600,#10601,#10602));
#3426=EDGE_LOOP('',(#10603,#10604,#10605));
#3427=EDGE_LOOP('',(#10606,#10607,#10608,#10609));
#3428=EDGE_LOOP('',(#10610,#10611,#10612));
#3429=EDGE_LOOP('',(#10613,#10614,#10615,#10616,#10617,#10618));
#3430=EDGE_LOOP('',(#10619,#10620,#10621));
#3431=EDGE_LOOP('',(#10622,#10623,#10624,#10625,#10626,#10627,#10628,#10629));
#3432=EDGE_LOOP('',(#10630,#10631,#10632,#10633,#10634,#10635));
#3433=EDGE_LOOP('',(#10636,#10637,#10638,#10639));
#3434=EDGE_LOOP('',(#10640,#10641,#10642,#10643));
#3435=EDGE_LOOP('',(#10644,#10645,#10646,#10647));
#3436=EDGE_LOOP('',(#10648,#10649,#10650,#10651));
#3437=EDGE_LOOP('',(#10652,#10653,#10654,#10655));
#3438=EDGE_LOOP('',(#10656,#10657,#10658,#10659));
#3439=EDGE_LOOP('',(#10660,#10661,#10662,#10663));
#3440=EDGE_LOOP('',(#10664,#10665,#10666,#10667));
#3441=EDGE_LOOP('',(#10668,#10669,#10670,#10671));
#3442=EDGE_LOOP('',(#10672,#10673,#10674,#10675));
#3443=EDGE_LOOP('',(#10676));
#3444=EDGE_LOOP('',(#10677,#10678,#10679,#10680,#10681,#10682));
#3445=EDGE_LOOP('',(#10683,#10684,#10685,#10686));
#3446=EDGE_LOOP('',(#10687,#10688,#10689,#10690));
#3447=EDGE_LOOP('',(#10691));
#3448=EDGE_LOOP('',(#10692,#10693,#10694,#10695,#10696,#10697,#10698,#10699,
#10700,#10701,#10702,#10703,#10704,#10705,#10706,#10707,#10708,#10709,#10710,
#10711));
#3449=EDGE_LOOP('',(#10712,#10713,#10714,#10715,#10716,#10717));
#3450=EDGE_LOOP('',(#10718));
#3451=EDGE_LOOP('',(#10719));
#3452=EDGE_LOOP('',(#10720));
#3453=EDGE_LOOP('',(#10721));
#3454=EDGE_LOOP('',(#10722));
#3455=EDGE_LOOP('',(#10723,#10724,#10725,#10726));
#3456=EDGE_LOOP('',(#10727));
#3457=EDGE_LOOP('',(#10728,#10729,#10730,#10731,#10732,#10733));
#3458=EDGE_LOOP('',(#10734,#10735,#10736,#10737,#10738,#10739,#10740,#10741));
#3459=EDGE_LOOP('',(#10742,#10743,#10744,#10745,#10746,#10747));
#3460=EDGE_LOOP('',(#10748,#10749,#10750,#10751,#10752,#10753,#10754,#10755));
#3461=EDGE_LOOP('',(#10756,#10757,#10758,#10759));
#3462=EDGE_LOOP('',(#10760));
#3463=EDGE_LOOP('',(#10761,#10762,#10763,#10764,#10765,#10766));
#3464=EDGE_LOOP('',(#10767,#10768,#10769,#10770));
#3465=EDGE_LOOP('',(#10771,#10772,#10773,#10774));
#3466=EDGE_LOOP('',(#10775,#10776,#10777,#10778));
#3467=EDGE_LOOP('',(#10779,#10780,#10781,#10782,#10783,#10784,#10785,#10786,
#10787,#10788,#10789,#10790,#10791,#10792,#10793,#10794));
#3468=EDGE_LOOP('',(#10795,#10796,#10797,#10798));
#3469=EDGE_LOOP('',(#10799,#10800,#10801,#10802));
#3470=EDGE_LOOP('',(#10803,#10804,#10805,#10806));
#3471=EDGE_LOOP('',(#10807,#10808,#10809,#10810));
#3472=EDGE_LOOP('',(#10811));
#3473=EDGE_LOOP('',(#10812));
#3474=EDGE_LOOP('',(#10813,#10814,#10815,#10816));
#3475=EDGE_LOOP('',(#10817));
#3476=EDGE_LOOP('',(#10818));
#3477=EDGE_LOOP('',(#10819,#10820,#10821,#10822));
#3478=EDGE_LOOP('',(#10823,#10824,#10825,#10826));
#3479=EDGE_LOOP('',(#10827,#10828,#10829,#10830));
#3480=EDGE_LOOP('',(#10831,#10832,#10833,#10834));
#3481=EDGE_LOOP('',(#10835,#10836,#10837,#10838));
#3482=EDGE_LOOP('',(#10839,#10840,#10841,#10842));
#3483=EDGE_LOOP('',(#10843,#10844,#10845,#10846));
#3484=EDGE_LOOP('',(#10847,#10848,#10849,#10850));
#3485=EDGE_LOOP('',(#10851,#10852,#10853,#10854));
#3486=EDGE_LOOP('',(#10855,#10856,#10857,#10858));
#3487=EDGE_LOOP('',(#10859,#10860,#10861,#10862));
#3488=EDGE_LOOP('',(#10863,#10864,#10865,#10866));
#3489=EDGE_LOOP('',(#10867,#10868,#10869,#10870));
#3490=EDGE_LOOP('',(#10871,#10872,#10873,#10874));
#3491=EDGE_LOOP('',(#10875,#10876,#10877,#10878));
#3492=EDGE_LOOP('',(#10879,#10880,#10881,#10882));
#3493=EDGE_LOOP('',(#10883,#10884,#10885,#10886));
#3494=EDGE_LOOP('',(#10887,#10888,#10889,#10890));
#3495=EDGE_LOOP('',(#10891,#10892,#10893,#10894));
#3496=EDGE_LOOP('',(#10895,#10896,#10897,#10898));
#3497=EDGE_LOOP('',(#10899,#10900,#10901,#10902));
#3498=EDGE_LOOP('',(#10903,#10904,#10905,#10906));
#3499=EDGE_LOOP('',(#10907,#10908,#10909,#10910));
#3500=EDGE_LOOP('',(#10911,#10912,#10913,#10914));
#3501=EDGE_LOOP('',(#10915,#10916,#10917,#10918));
#3502=EDGE_LOOP('',(#10919,#10920,#10921,#10922));
#3503=EDGE_LOOP('',(#10923,#10924,#10925,#10926));
#3504=EDGE_LOOP('',(#10927,#10928,#10929,#10930));
#3505=EDGE_LOOP('',(#10931,#10932,#10933,#10934));
#3506=EDGE_LOOP('',(#10935,#10936,#10937,#10938));
#3507=EDGE_LOOP('',(#10939,#10940,#10941,#10942));
#3508=EDGE_LOOP('',(#10943));
#3509=EDGE_LOOP('',(#10944));
#3510=EDGE_LOOP('',(#10945,#10946,#10947,#10948));
#3511=EDGE_LOOP('',(#10949));
#3512=EDGE_LOOP('',(#10950));
#3513=EDGE_LOOP('',(#10951,#10952,#10953,#10954));
#3514=EDGE_LOOP('',(#10955));
#3515=EDGE_LOOP('',(#10956));
#3516=EDGE_LOOP('',(#10957,#10958,#10959,#10960,#10961,#10962,#10963,#10964,
#10965));
#3517=EDGE_LOOP('',(#10966,#10967));
#3518=EDGE_LOOP('',(#10968));
#3519=EDGE_LOOP('',(#10969));
#3520=EDGE_LOOP('',(#10970,#10971,#10972,#10973));
#3521=EDGE_LOOP('',(#10974));
#3522=EDGE_LOOP('',(#10975));
#3523=EDGE_LOOP('',(#10976,#10977,#10978,#10979));
#3524=EDGE_LOOP('',(#10980));
#3525=EDGE_LOOP('',(#10981));
#3526=EDGE_LOOP('',(#10982,#10983,#10984,#10985));
#3527=EDGE_LOOP('',(#10986,#10987,#10988,#10989));
#3528=EDGE_LOOP('',(#10990,#10991,#10992));
#3529=EDGE_LOOP('',(#10993));
#3530=EDGE_LOOP('',(#10994));
#3531=EDGE_LOOP('',(#10995,#10996,#10997,#10998));
#3532=EDGE_LOOP('',(#10999));
#3533=EDGE_LOOP('',(#11000));
#3534=EDGE_LOOP('',(#11001,#11002,#11003,#11004));
#3535=EDGE_LOOP('',(#11005,#11006,#11007,#11008));
#3536=EDGE_LOOP('',(#11009,#11010,#11011,#11012));
#3537=EDGE_LOOP('',(#11013,#11014,#11015,#11016));
#3538=EDGE_LOOP('',(#11017,#11018,#11019,#11020));
#4281=LINE('',#21063,#5141);
#4282=LINE('',#21065,#5142);
#4283=LINE('',#21067,#5143);
#4284=LINE('',#21068,#5144);
#4285=LINE('',#21071,#5145);
#4286=LINE('',#21073,#5146);
#4287=LINE('',#21074,#5147);
#4288=LINE('',#21077,#5148);
#4289=LINE('',#21079,#5149);
#4290=LINE('',#21080,#5150);
#4291=LINE('',#21082,#5151);
#4292=LINE('',#21083,#5152);
#4293=LINE('',#21088,#5153);
#4294=LINE('',#21090,#5154);
#4295=LINE('',#21092,#5155);
#4296=LINE('',#21093,#5156);
#4297=LINE('',#21096,#5157);
#4298=LINE('',#21098,#5158);
#4299=LINE('',#21100,#5159);
#4300=LINE('',#21102,#5160);
#4301=LINE('',#21103,#5161);
#4302=LINE('',#21106,#5162);
#4303=LINE('',#21107,#5163);
#4304=LINE('',#21110,#5164);
#4305=LINE('',#21111,#5165);
#4306=LINE('',#21114,#5166);
#4307=LINE('',#21115,#5167);
#4308=LINE('',#21119,#5168);
#4309=LINE('',#21121,#5169);
#4310=LINE('',#21123,#5170);
#4311=LINE('',#21124,#5171);
#4312=LINE('',#21127,#5172);
#4313=LINE('',#21129,#5173);
#4314=LINE('',#21130,#5174);
#4315=LINE('',#21133,#5175);
#4316=LINE('',#21135,#5176);
#4317=LINE('',#21136,#5177);
#4318=LINE('',#21138,#5178);
#4319=LINE('',#21139,#5179);
#4320=LINE('',#21144,#5180);
#4321=LINE('',#21146,#5181);
#4322=LINE('',#21148,#5182);
#4323=LINE('',#21149,#5183);
#4324=LINE('',#21152,#5184);
#4325=LINE('',#21154,#5185);
#4326=LINE('',#21155,#5186);
#4327=LINE('',#21158,#5187);
#4328=LINE('',#21160,#5188);
#4329=LINE('',#21161,#5189);
#4330=LINE('',#21163,#5190);
#4331=LINE('',#21164,#5191);
#4332=LINE('',#21169,#5192);
#4333=LINE('',#21171,#5193);
#4334=LINE('',#21173,#5194);
#4335=LINE('',#21174,#5195);
#4336=LINE('',#21177,#5196);
#4337=LINE('',#21179,#5197);
#4338=LINE('',#21180,#5198);
#4339=LINE('',#21183,#5199);
#4340=LINE('',#21185,#5200);
#4341=LINE('',#21186,#5201);
#4342=LINE('',#21188,#5202);
#4343=LINE('',#21189,#5203);
#4344=LINE('',#21194,#5204);
#4345=LINE('',#21196,#5205);
#4346=LINE('',#21198,#5206);
#4347=LINE('',#21199,#5207);
#4348=LINE('',#21203,#5208);
#4349=LINE('',#21205,#5209);
#4350=LINE('',#21207,#5210);
#4351=LINE('',#21208,#5211);
#4352=LINE('',#21211,#5212);
#4353=LINE('',#21213,#5213);
#4354=LINE('',#21214,#5214);
#4355=LINE('',#21216,#5215);
#4356=LINE('',#21217,#5216);
#4357=LINE('',#21220,#5217);
#4358=LINE('',#21221,#5218);
#4359=LINE('',#21224,#5219);
#4360=LINE('',#21226,#5220);
#4361=LINE('',#21228,#5221);
#4362=LINE('',#21229,#5222);
#4363=LINE('',#21232,#5223);
#4364=LINE('',#21234,#5224);
#4365=LINE('',#21235,#5225);
#4366=LINE('',#21238,#5226);
#4367=LINE('',#21240,#5227);
#4368=LINE('',#21242,#5228);
#4369=LINE('',#21244,#5229);
#4370=LINE('',#21246,#5230);
#4371=LINE('',#21247,#5231);
#4372=LINE('',#21249,#5232);
#4373=LINE('',#21251,#5233);
#4374=LINE('',#21253,#5234);
#4375=LINE('',#21254,#5235);
#4376=LINE('',#21260,#5236);
#4377=LINE('',#21262,#5237);
#4378=LINE('',#21264,#5238);
#4379=LINE('',#21265,#5239);
#4380=LINE('',#21268,#5240);
#4381=LINE('',#21270,#5241);
#4382=LINE('',#21271,#5242);
#4383=LINE('',#21274,#5243);
#4384=LINE('',#21276,#5244);
#4385=LINE('',#21277,#5245);
#4386=LINE('',#21279,#5246);
#4387=LINE('',#21280,#5247);
#4388=LINE('',#21285,#5248);
#4389=LINE('',#21287,#5249);
#4390=LINE('',#21289,#5250);
#4391=LINE('',#21290,#5251);
#4392=LINE('',#21294,#5252);
#4393=LINE('',#21296,#5253);
#4394=LINE('',#21298,#5254);
#4395=LINE('',#21299,#5255);
#4396=LINE('',#21301,#5256);
#4397=LINE('',#21302,#5257);
#4398=LINE('',#21306,#5258);
#4399=LINE('',#21307,#5259);
#4400=LINE('',#21308,#5260);
#4401=LINE('',#21311,#5261);
#4402=LINE('',#21312,#5262);
#4403=LINE('',#21316,#5263);
#4404=LINE('',#21318,#5264);
#4405=LINE('',#21320,#5265);
#4406=LINE('',#21321,#5266);
#4407=LINE('',#21324,#5267);
#4408=LINE('',#21326,#5268);
#4409=LINE('',#21327,#5269);
#4410=LINE('',#21330,#5270);
#4411=LINE('',#21332,#5271);
#4412=LINE('',#21333,#5272);
#4413=LINE('',#21335,#5273);
#4414=LINE('',#21336,#5274);
#4415=LINE('',#21341,#5275);
#4416=LINE('',#21343,#5276);
#4417=LINE('',#21345,#5277);
#4418=LINE('',#21346,#5278);
#4419=LINE('',#21349,#5279);
#4420=LINE('',#21351,#5280);
#4421=LINE('',#21352,#5281);
#4422=LINE('',#21355,#5282);
#4423=LINE('',#21357,#5283);
#4424=LINE('',#21358,#5284);
#4425=LINE('',#21360,#5285);
#4426=LINE('',#21361,#5286);
#4427=LINE('',#21366,#5287);
#4428=LINE('',#21368,#5288);
#4429=LINE('',#21370,#5289);
#4430=LINE('',#21371,#5290);
#4431=LINE('',#21374,#5291);
#4432=LINE('',#21376,#5292);
#4433=LINE('',#21377,#5293);
#4434=LINE('',#21380,#5294);
#4435=LINE('',#21382,#5295);
#4436=LINE('',#21383,#5296);
#4437=LINE('',#21385,#5297);
#4438=LINE('',#21386,#5298);
#4439=LINE('',#21391,#5299);
#4440=LINE('',#21393,#5300);
#4441=LINE('',#21395,#5301);
#4442=LINE('',#21396,#5302);
#4443=LINE('',#21399,#5303);
#4444=LINE('',#21401,#5304);
#4445=LINE('',#21402,#5305);
#4446=LINE('',#21406,#5306);
#4447=LINE('',#21408,#5307);
#4448=LINE('',#21410,#5308);
#4449=LINE('',#21411,#5309);
#4450=LINE('',#21413,#5310);
#4451=LINE('',#21414,#5311);
#4452=LINE('',#21417,#5312);
#4453=LINE('',#21418,#5313);
#4454=LINE('',#21421,#5314);
#4455=LINE('',#21423,#5315);
#4456=LINE('',#21425,#5316);
#4457=LINE('',#21426,#5317);
#4458=LINE('',#21429,#5318);
#4459=LINE('',#21431,#5319);
#4460=LINE('',#21433,#5320);
#4461=LINE('',#21434,#5321);
#4462=LINE('',#21437,#5322);
#4463=LINE('',#21439,#5323);
#4464=LINE('',#21441,#5324);
#4465=LINE('',#21447,#5325);
#4466=LINE('',#21453,#5326);
#4467=LINE('',#21454,#5327);
#4468=LINE('',#21456,#5328);
#4469=LINE('',#21458,#5329);
#4470=LINE('',#21460,#5330);
#4471=LINE('',#21462,#5331);
#4472=LINE('',#21464,#5332);
#4473=LINE('',#21465,#5333);
#4474=LINE('',#21477,#5334);
#4475=LINE('',#21480,#5335);
#4476=LINE('',#21485,#5336);
#4477=LINE('',#21489,#5337);
#4478=LINE('',#21491,#5338);
#4479=LINE('',#21492,#5339);
#4480=LINE('',#21495,#5340);
#4481=LINE('',#21497,#5341);
#4482=LINE('',#21498,#5342);
#4483=LINE('',#21501,#5343);
#4484=LINE('',#21503,#5344);
#4485=LINE('',#21504,#5345);
#4486=LINE('',#21512,#5346);
#4487=LINE('',#21514,#5347);
#4488=LINE('',#21516,#5348);
#4489=LINE('',#21517,#5349);
#4490=LINE('',#21520,#5350);
#4491=LINE('',#21522,#5351);
#4492=LINE('',#21523,#5352);
#4493=LINE('',#21526,#5353);
#4494=LINE('',#21528,#5354);
#4495=LINE('',#21529,#5355);
#4496=LINE('',#21543,#5356);
#4497=LINE('',#21547,#5357);
#4498=LINE('',#21550,#5358);
#4499=LINE('',#21552,#5359);
#4500=LINE('',#21581,#5360);
#4501=LINE('',#21584,#5361);
#4502=LINE('',#21611,#5362);
#4503=LINE('',#21614,#5363);
#4504=LINE('',#21655,#5364);
#4505=LINE('',#21656,#5365);
#4506=LINE('',#21658,#5366);
#4507=LINE('',#21660,#5367);
#4508=LINE('',#21662,#5368);
#4509=LINE('',#21664,#5369);
#4510=LINE('',#21666,#5370);
#4511=LINE('',#21718,#5371);
#4512=LINE('',#21722,#5372);
#4513=LINE('',#21727,#5373);
#4514=LINE('',#21731,#5374);
#4515=LINE('',#21763,#5375);
#4516=LINE('',#21794,#5376);
#4517=LINE('',#21811,#5377);
#4518=LINE('',#21813,#5378);
#4519=LINE('',#21815,#5379);
#4520=LINE('',#21821,#5380);
#4521=LINE('',#21826,#5381);
#4522=LINE('',#21828,#5382);
#4523=LINE('',#21833,#5383);
#4524=LINE('',#21836,#5384);
#4525=LINE('',#21838,#5385);
#4526=LINE('',#21840,#5386);
#4527=LINE('',#21841,#5387);
#4528=LINE('',#21844,#5388);
#4529=LINE('',#21846,#5389);
#4530=LINE('',#21848,#5390);
#4531=LINE('',#21849,#5391);
#4532=LINE('',#21852,#5392);
#4533=LINE('',#21854,#5393);
#4534=LINE('',#21856,#5394);
#4535=LINE('',#21857,#5395);
#4536=LINE('',#21860,#5396);
#4537=LINE('',#21862,#5397);
#4538=LINE('',#21864,#5398);
#4539=LINE('',#21865,#5399);
#4540=LINE('',#21868,#5400);
#4541=LINE('',#21870,#5401);
#4542=LINE('',#21872,#5402);
#4543=LINE('',#21873,#5403);
#4544=LINE('',#21876,#5404);
#4545=LINE('',#21878,#5405);
#4546=LINE('',#21880,#5406);
#4547=LINE('',#21881,#5407);
#4548=LINE('',#21885,#5408);
#4549=LINE('',#21889,#5409);
#4550=LINE('',#21946,#5410);
#4551=LINE('',#22008,#5411);
#4552=LINE('',#22012,#5412);
#4553=LINE('',#22015,#5413);
#4554=LINE('',#22041,#5414);
#4555=LINE('',#22045,#5415);
#4556=LINE('',#22048,#5416);
#4557=LINE('',#22052,#5417);
#4558=LINE('',#22056,#5418);
#4559=LINE('',#22059,#5419);
#4560=LINE('',#22063,#5420);
#4561=LINE('',#22067,#5421);
#4562=LINE('',#22071,#5422);
#4563=LINE('',#22076,#5423);
#4564=LINE('',#22080,#5424);
#4565=LINE('',#22083,#5425);
#4566=LINE('',#22087,#5426);
#4567=LINE('',#22091,#5427);
#4568=LINE('',#22095,#5428);
#4569=LINE('',#22100,#5429);
#4570=LINE('',#22104,#5430);
#4571=LINE('',#22107,#5431);
#4572=LINE('',#22111,#5432);
#4573=LINE('',#22115,#5433);
#4574=LINE('',#22119,#5434);
#4575=LINE('',#22124,#5435);
#4576=LINE('',#22128,#5436);
#4577=LINE('',#22131,#5437);
#4578=LINE('',#22135,#5438);
#4579=LINE('',#22139,#5439);
#4580=LINE('',#22143,#5440);
#4581=LINE('',#22148,#5441);
#4582=LINE('',#22152,#5442);
#4583=LINE('',#22155,#5443);
#4584=LINE('',#22159,#5444);
#4585=LINE('',#22163,#5445);
#4586=LINE('',#22166,#5446);
#4587=LINE('',#22170,#5447);
#4588=LINE('',#22174,#5448);
#4589=LINE('',#22177,#5449);
#4590=LINE('',#22181,#5450);
#4591=LINE('',#22184,#5451);
#4592=LINE('',#22186,#5452);
#4593=LINE('',#22189,#5453);
#4594=LINE('',#22194,#5454);
#4595=LINE('',#22198,#5455);
#4596=LINE('',#22204,#5456);
#4597=LINE('',#22208,#5457);
#4598=LINE('',#22214,#5458);
#4599=LINE('',#22218,#5459);
#4600=LINE('',#22224,#5460);
#4601=LINE('',#22228,#5461);
#4602=LINE('',#22232,#5462);
#4603=LINE('',#22233,#5463);
#4604=LINE('',#22235,#5464);
#4605=LINE('',#22238,#5465);
#4606=LINE('',#22239,#5466);
#4607=LINE('',#22242,#5467);
#4608=LINE('',#22243,#5468);
#4609=LINE('',#22245,#5469);
#4610=LINE('',#22250,#5470);
#4611=LINE('',#22252,#5471);
#4612=LINE('',#22254,#5472);
#4613=LINE('',#22256,#5473);
#4614=LINE('',#22258,#5474);
#4615=LINE('',#22264,#5475);
#4616=LINE('',#22266,#5476);
#4617=LINE('',#22267,#5477);
#4618=LINE('',#22270,#5478);
#4619=LINE('',#22271,#5479);
#4620=LINE('',#22273,#5480);
#4621=LINE('',#22275,#5481);
#4622=LINE('',#22276,#5482);
#4623=LINE('',#22280,#5483);
#4624=LINE('',#22282,#5484);
#4625=LINE('',#22284,#5485);
#4626=LINE('',#22285,#5486);
#4627=LINE('',#22286,#5487);
#4628=LINE('',#22288,#5488);
#4629=LINE('',#22289,#5489);
#4630=LINE('',#22294,#5490);
#4631=LINE('',#22298,#5491);
#4632=LINE('',#22304,#5492);
#4633=LINE('',#22306,#5493);
#4634=LINE('',#22308,#5494);
#4635=LINE('',#22310,#5495);
#4636=LINE('',#22312,#5496);
#4637=LINE('',#22316,#5497);
#4638=LINE('',#22317,#5498);
#4639=LINE('',#22319,#5499);
#4640=LINE('',#22320,#5500);
#4641=LINE('',#22323,#5501);
#4642=LINE('',#22325,#5502);
#4643=LINE('',#22328,#5503);
#4644=LINE('',#22330,#5504);
#4645=LINE('',#22331,#5505);
#4646=LINE('',#22334,#5506);
#4647=LINE('',#22335,#5507);
#4648=LINE('',#22338,#5508);
#4649=LINE('',#22339,#5509);
#4650=LINE('',#22341,#5510);
#4651=LINE('',#22345,#5511);
#4652=LINE('',#22347,#5512);
#4653=LINE('',#22348,#5513);
#4654=LINE('',#22351,#5514);
#4655=LINE('',#22352,#5515);
#4656=LINE('',#22355,#5516);
#4657=LINE('',#22356,#5517);
#4658=LINE('',#22358,#5518);
#4659=LINE('',#22362,#5519);
#4660=LINE('',#22364,#5520);
#4661=LINE('',#22365,#5521);
#4662=LINE('',#22368,#5522);
#4663=LINE('',#22369,#5523);
#4664=LINE('',#22372,#5524);
#4665=LINE('',#22373,#5525);
#4666=LINE('',#22375,#5526);
#4667=LINE('',#22379,#5527);
#4668=LINE('',#22381,#5528);
#4669=LINE('',#22382,#5529);
#4670=LINE('',#22385,#5530);
#4671=LINE('',#22386,#5531);
#4672=LINE('',#22389,#5532);
#4673=LINE('',#22390,#5533);
#4674=LINE('',#22392,#5534);
#4675=LINE('',#22396,#5535);
#4676=LINE('',#22398,#5536);
#4677=LINE('',#22399,#5537);
#4678=LINE('',#22402,#5538);
#4679=LINE('',#22403,#5539);
#4680=LINE('',#22406,#5540);
#4681=LINE('',#22407,#5541);
#4682=LINE('',#22409,#5542);
#4683=LINE('',#22413,#5543);
#4684=LINE('',#22415,#5544);
#4685=LINE('',#22416,#5545);
#4686=LINE('',#22419,#5546);
#4687=LINE('',#22420,#5547);
#4688=LINE('',#22423,#5548);
#4689=LINE('',#22424,#5549);
#4690=LINE('',#22426,#5550);
#4691=LINE('',#22430,#5551);
#4692=LINE('',#22437,#5552);
#4693=LINE('',#22444,#5553);
#4694=LINE('',#22451,#5554);
#4695=LINE('',#22491,#5555);
#4696=LINE('',#22533,#5556);
#4697=LINE('',#22540,#5557);
#4698=LINE('',#22546,#5558);
#4699=LINE('',#22549,#5559);
#4700=LINE('',#22556,#5560);
#4701=LINE('',#22563,#5561);
#4702=LINE('',#22566,#5562);
#5141=VECTOR('',#17292,1.);
#5142=VECTOR('',#17293,1.);
#5143=VECTOR('',#17294,1.);
#5144=VECTOR('',#17295,1.);
#5145=VECTOR('',#17298,1.);
#5146=VECTOR('',#17299,1.);
#5147=VECTOR('',#17300,1.);
#5148=VECTOR('',#17303,1.);
#5149=VECTOR('',#17304,1.);
#5150=VECTOR('',#17305,1.);
#5151=VECTOR('',#17308,1.);
#5152=VECTOR('',#17309,1.);
#5153=VECTOR('',#17314,1.);
#5154=VECTOR('',#17315,1.);
#5155=VECTOR('',#17316,1.);
#5156=VECTOR('',#17317,1.);
#5157=VECTOR('',#17320,1.);
#5158=VECTOR('',#17321,1.);
#5159=VECTOR('',#17322,1.);
#5160=VECTOR('',#17323,1.);
#5161=VECTOR('',#17324,1.);
#5162=VECTOR('',#17327,1.);
#5163=VECTOR('',#17328,1.);
#5164=VECTOR('',#17331,1.);
#5165=VECTOR('',#17332,1.);
#5166=VECTOR('',#17335,1.);
#5167=VECTOR('',#17336,1.);
#5168=VECTOR('',#17339,1.);
#5169=VECTOR('',#17340,1.);
#5170=VECTOR('',#17341,1.);
#5171=VECTOR('',#17342,1.);
#5172=VECTOR('',#17345,1.);
#5173=VECTOR('',#17346,1.);
#5174=VECTOR('',#17347,1.);
#5175=VECTOR('',#17350,1.);
#5176=VECTOR('',#17351,1.);
#5177=VECTOR('',#17352,1.);
#5178=VECTOR('',#17355,1.);
#5179=VECTOR('',#17356,1.);
#5180=VECTOR('',#17361,1.);
#5181=VECTOR('',#17362,1.);
#5182=VECTOR('',#17363,1.);
#5183=VECTOR('',#17364,1.);
#5184=VECTOR('',#17367,1.);
#5185=VECTOR('',#17368,1.);
#5186=VECTOR('',#17369,1.);
#5187=VECTOR('',#17372,1.);
#5188=VECTOR('',#17373,1.);
#5189=VECTOR('',#17374,1.);
#5190=VECTOR('',#17377,1.);
#5191=VECTOR('',#17378,1.);
#5192=VECTOR('',#17383,1.);
#5193=VECTOR('',#17384,1.);
#5194=VECTOR('',#17385,1.);
#5195=VECTOR('',#17386,1.);
#5196=VECTOR('',#17389,1.);
#5197=VECTOR('',#17390,1.);
#5198=VECTOR('',#17391,1.);
#5199=VECTOR('',#17394,1.);
#5200=VECTOR('',#17395,1.);
#5201=VECTOR('',#17396,1.);
#5202=VECTOR('',#17399,1.);
#5203=VECTOR('',#17400,1.);
#5204=VECTOR('',#17405,1.);
#5205=VECTOR('',#17406,1.);
#5206=VECTOR('',#17407,1.);
#5207=VECTOR('',#17408,1.);
#5208=VECTOR('',#17411,1.);
#5209=VECTOR('',#17412,1.);
#5210=VECTOR('',#17413,1.);
#5211=VECTOR('',#17414,1.);
#5212=VECTOR('',#17417,1.);
#5213=VECTOR('',#17418,1.);
#5214=VECTOR('',#17419,1.);
#5215=VECTOR('',#17422,1.);
#5216=VECTOR('',#17423,1.);
#5217=VECTOR('',#17426,1.);
#5218=VECTOR('',#17427,1.);
#5219=VECTOR('',#17430,1.);
#5220=VECTOR('',#17431,1.);
#5221=VECTOR('',#17432,1.);
#5222=VECTOR('',#17433,1.);
#5223=VECTOR('',#17436,1.);
#5224=VECTOR('',#17437,1.);
#5225=VECTOR('',#17438,1.);
#5226=VECTOR('',#17441,1.);
#5227=VECTOR('',#17442,1.);
#5228=VECTOR('',#17443,1.);
#5229=VECTOR('',#17444,1.);
#5230=VECTOR('',#17445,1.);
#5231=VECTOR('',#17446,1.);
#5232=VECTOR('',#17447,1.);
#5233=VECTOR('',#17448,1.);
#5234=VECTOR('',#17449,1.);
#5235=VECTOR('',#17450,1.);
#5236=VECTOR('',#17455,1.);
#5237=VECTOR('',#17456,1.);
#5238=VECTOR('',#17457,1.);
#5239=VECTOR('',#17458,1.);
#5240=VECTOR('',#17461,1.);
#5241=VECTOR('',#17462,1.);
#5242=VECTOR('',#17463,1.);
#5243=VECTOR('',#17466,1.);
#5244=VECTOR('',#17467,1.);
#5245=VECTOR('',#17468,1.);
#5246=VECTOR('',#17471,1.);
#5247=VECTOR('',#17472,1.);
#5248=VECTOR('',#17477,1.);
#5249=VECTOR('',#17478,1.);
#5250=VECTOR('',#17479,1.);
#5251=VECTOR('',#17480,1.);
#5252=VECTOR('',#17483,1.);
#5253=VECTOR('',#17484,1.);
#5254=VECTOR('',#17485,1.);
#5255=VECTOR('',#17486,1.);
#5256=VECTOR('',#17489,1.);
#5257=VECTOR('',#17490,1.);
#5258=VECTOR('',#17493,1.);
#5259=VECTOR('',#17494,1.);
#5260=VECTOR('',#17495,1.);
#5261=VECTOR('',#17498,1.);
#5262=VECTOR('',#17499,1.);
#5263=VECTOR('',#17502,1.);
#5264=VECTOR('',#17503,1.);
#5265=VECTOR('',#17504,1.);
#5266=VECTOR('',#17505,1.);
#5267=VECTOR('',#17508,1.);
#5268=VECTOR('',#17509,1.);
#5269=VECTOR('',#17510,1.);
#5270=VECTOR('',#17513,1.);
#5271=VECTOR('',#17514,1.);
#5272=VECTOR('',#17515,1.);
#5273=VECTOR('',#17518,1.);
#5274=VECTOR('',#17519,1.);
#5275=VECTOR('',#17524,1.);
#5276=VECTOR('',#17525,1.);
#5277=VECTOR('',#17526,1.);
#5278=VECTOR('',#17527,1.);
#5279=VECTOR('',#17530,1.);
#5280=VECTOR('',#17531,1.);
#5281=VECTOR('',#17532,1.);
#5282=VECTOR('',#17535,1.);
#5283=VECTOR('',#17536,1.);
#5284=VECTOR('',#17537,1.);
#5285=VECTOR('',#17540,1.);
#5286=VECTOR('',#17541,1.);
#5287=VECTOR('',#17546,1.);
#5288=VECTOR('',#17547,1.);
#5289=VECTOR('',#17548,1.);
#5290=VECTOR('',#17549,1.);
#5291=VECTOR('',#17552,1.);
#5292=VECTOR('',#17553,1.);
#5293=VECTOR('',#17554,1.);
#5294=VECTOR('',#17557,1.);
#5295=VECTOR('',#17558,1.);
#5296=VECTOR('',#17559,1.);
#5297=VECTOR('',#17562,1.);
#5298=VECTOR('',#17563,1.);
#5299=VECTOR('',#17568,1.);
#5300=VECTOR('',#17569,1.);
#5301=VECTOR('',#17570,1.);
#5302=VECTOR('',#17571,1.);
#5303=VECTOR('',#17574,1.);
#5304=VECTOR('',#17575,1.);
#5305=VECTOR('',#17576,1.);
#5306=VECTOR('',#17579,1.);
#5307=VECTOR('',#17580,1.);
#5308=VECTOR('',#17581,1.);
#5309=VECTOR('',#17582,1.);
#5310=VECTOR('',#17585,1.);
#5311=VECTOR('',#17586,1.);
#5312=VECTOR('',#17589,1.);
#5313=VECTOR('',#17590,1.);
#5314=VECTOR('',#17593,1.);
#5315=VECTOR('',#17594,1.);
#5316=VECTOR('',#17595,1.);
#5317=VECTOR('',#17596,1.);
#5318=VECTOR('',#17599,1.);
#5319=VECTOR('',#17600,1.);
#5320=VECTOR('',#17601,1.);
#5321=VECTOR('',#17602,1.);
#5322=VECTOR('',#17605,1.);
#5323=VECTOR('',#17606,1.);
#5324=VECTOR('',#17607,1.);
#5325=VECTOR('',#17612,1.);
#5326=VECTOR('',#17617,1.);
#5327=VECTOR('',#17618,1.);
#5328=VECTOR('',#17619,1.);
#5329=VECTOR('',#17620,1.);
#5330=VECTOR('',#17621,1.);
#5331=VECTOR('',#17622,1.);
#5332=VECTOR('',#17623,1.);
#5333=VECTOR('',#17624,1.);
#5334=VECTOR('',#17635,1.);
#5335=VECTOR('',#17638,1.);
#5336=VECTOR('',#17643,1.);
#5337=VECTOR('',#17648,1.);
#5338=VECTOR('',#17649,1.);
#5339=VECTOR('',#17650,1.);
#5340=VECTOR('',#17653,1.);
#5341=VECTOR('',#17654,1.);
#5342=VECTOR('',#17655,1.);
#5343=VECTOR('',#17658,1.);
#5344=VECTOR('',#17659,1.);
#5345=VECTOR('',#17660,1.);
#5346=VECTOR('',#17671,1.);
#5347=VECTOR('',#17672,1.);
#5348=VECTOR('',#17673,1.);
#5349=VECTOR('',#17674,1.);
#5350=VECTOR('',#17677,1.);
#5351=VECTOR('',#17678,1.);
#5352=VECTOR('',#17679,1.);
#5353=VECTOR('',#17682,1.);
#5354=VECTOR('',#17683,1.);
#5355=VECTOR('',#17684,1.);
#5356=VECTOR('',#17701,1.);
#5357=VECTOR('',#17704,1.);
#5358=VECTOR('',#17707,1.);
#5359=VECTOR('',#17708,1.);
#5360=VECTOR('',#17731,1.);
#5361=VECTOR('',#17734,1.);
#5362=VECTOR('',#17757,1.);
#5363=VECTOR('',#17760,1.);
#5364=VECTOR('',#17793,1.);
#5365=VECTOR('',#17794,1.);
#5366=VECTOR('',#17797,1.);
#5367=VECTOR('',#17800,1.);
#5368=VECTOR('',#17803,1.);
#5369=VECTOR('',#17806,1.);
#5370=VECTOR('',#17809,1.);
#5371=VECTOR('',#17824,0.505);
#5372=VECTOR('',#17829,0.5575);
#5373=VECTOR('',#17834,0.2025);
#5374=VECTOR('',#17839,0.405);
#5375=VECTOR('',#17840,0.405);
#5376=VECTOR('',#17845,0.455);
#5377=VECTOR('',#17852,1.);
#5378=VECTOR('',#17853,1.);
#5379=VECTOR('',#17854,1.);
#5380=VECTOR('',#17859,1.);
#5381=VECTOR('',#17864,1.);
#5382=VECTOR('',#17865,1.);
#5383=VECTOR('',#17870,1.);
#5384=VECTOR('',#17871,1.);
#5385=VECTOR('',#17872,1.);
#5386=VECTOR('',#17873,1.);
#5387=VECTOR('',#17874,1.);
#5388=VECTOR('',#17875,1.);
#5389=VECTOR('',#17876,1.);
#5390=VECTOR('',#17877,1.);
#5391=VECTOR('',#17878,1.);
#5392=VECTOR('',#17879,1.);
#5393=VECTOR('',#17880,1.);
#5394=VECTOR('',#17881,1.);
#5395=VECTOR('',#17882,1.);
#5396=VECTOR('',#17883,1.);
#5397=VECTOR('',#17884,1.);
#5398=VECTOR('',#17885,1.);
#5399=VECTOR('',#17886,1.);
#5400=VECTOR('',#17887,1.);
#5401=VECTOR('',#17888,1.);
#5402=VECTOR('',#17889,1.);
#5403=VECTOR('',#17890,1.);
#5404=VECTOR('',#17891,1.);
#5405=VECTOR('',#17892,1.);
#5406=VECTOR('',#17893,1.);
#5407=VECTOR('',#17894,1.);
#5408=VECTOR('',#17897,0.2025);
#5409=VECTOR('',#17902,0.405);
#5410=VECTOR('',#17907,0.455000000000001);
#5411=VECTOR('',#17914,0.2025);
#5412=VECTOR('',#17919,0.405);
#5413=VECTOR('',#17924,0.455);
#5414=VECTOR('',#17931,0.2025);
#5415=VECTOR('',#17936,0.405);
#5416=VECTOR('',#17941,0.455000000000001);
#5417=VECTOR('',#17944,0.1525);
#5418=VECTOR('',#17949,0.305);
#5419=VECTOR('',#17954,0.355);
#5420=VECTOR('',#17957,0.1525);
#5421=VECTOR('',#17962,0.305);
#5422=VECTOR('',#17967,0.355);
#5423=VECTOR('',#17972,0.1525);
#5424=VECTOR('',#17977,0.305);
#5425=VECTOR('',#17982,0.355);
#5426=VECTOR('',#17985,0.1525);
#5427=VECTOR('',#17990,0.305);
#5428=VECTOR('',#17995,0.355);
#5429=VECTOR('',#18000,0.1525);
#5430=VECTOR('',#18005,0.305);
#5431=VECTOR('',#18010,0.355);
#5432=VECTOR('',#18013,0.1525);
#5433=VECTOR('',#18018,0.305);
#5434=VECTOR('',#18023,0.355);
#5435=VECTOR('',#18028,0.1525);
#5436=VECTOR('',#18033,0.305);
#5437=VECTOR('',#18038,0.355);
#5438=VECTOR('',#18041,0.1525);
#5439=VECTOR('',#18046,0.305);
#5440=VECTOR('',#18051,0.355);
#5441=VECTOR('',#18056,0.1525);
#5442=VECTOR('',#18061,0.305);
#5443=VECTOR('',#18066,0.355);
#5444=VECTOR('',#18069,0.1525);
#5445=VECTOR('',#18074,0.305);
#5446=VECTOR('',#18079,0.355);
#5447=VECTOR('',#18082,0.1525);
#5448=VECTOR('',#18087,0.305);
#5449=VECTOR('',#18092,0.355);
#5450=VECTOR('',#18095,0.1525);
#5451=VECTOR('',#18100,0.305);
#5452=VECTOR('',#18101,0.305);
#5453=VECTOR('',#18106,0.355);
#5454=VECTOR('',#18111,0.425);
#5455=VECTOR('',#18116,0.462499999999999);
#5456=VECTOR('',#18123,0.425000000000001);
#5457=VECTOR('',#18128,0.4625);
#5458=VECTOR('',#18135,0.425);
#5459=VECTOR('',#18140,0.462499999999999);
#5460=VECTOR('',#18147,0.425000000000001);
#5461=VECTOR('',#18152,0.4625);
#5462=VECTOR('',#18157,1.);
#5463=VECTOR('',#18158,1.);
#5464=VECTOR('',#18161,1.);
#5465=VECTOR('',#18164,1.);
#5466=VECTOR('',#18165,1.);
#5467=VECTOR('',#18168,1.);
#5468=VECTOR('',#18169,1.);
#5469=VECTOR('',#18172,1.);
#5470=VECTOR('',#18177,1.);
#5471=VECTOR('',#18178,1.);
#5472=VECTOR('',#18179,1.);
#5473=VECTOR('',#18180,1.);
#5474=VECTOR('',#18181,1.);
#5475=VECTOR('',#18188,1.);
#5476=VECTOR('',#18189,1.);
#5477=VECTOR('',#18190,1.);
#5478=VECTOR('',#18193,1.);
#5479=VECTOR('',#18194,1.);
#5480=VECTOR('',#18197,1.);
#5481=VECTOR('',#18198,1.);
#5482=VECTOR('',#18199,1.);
#5483=VECTOR('',#18204,1.);
#5484=VECTOR('',#18205,1.);
#5485=VECTOR('',#18206,1.);
#5486=VECTOR('',#18207,1.);
#5487=VECTOR('',#18208,1.);
#5488=VECTOR('',#18211,1.);
#5489=VECTOR('',#18212,1.);
#5490=VECTOR('',#18219,1.);
#5491=VECTOR('',#18224,1.);
#5492=VECTOR('',#18231,1.);
#5493=VECTOR('',#18232,1.);
#5494=VECTOR('',#18233,1.);
#5495=VECTOR('',#18234,1.);
#5496=VECTOR('',#18235,1.);
#5497=VECTOR('',#18242,1.);
#5498=VECTOR('',#18243,1.);
#5499=VECTOR('',#18246,1.);
#5500=VECTOR('',#18247,1.);
#5501=VECTOR('',#18252,1.);
#5502=VECTOR('',#18255,1.);
#5503=VECTOR('',#18258,1.);
#5504=VECTOR('',#18259,1.);
#5505=VECTOR('',#18260,1.);
#5506=VECTOR('',#18263,1.);
#5507=VECTOR('',#18264,1.);
#5508=VECTOR('',#18267,1.);
#5509=VECTOR('',#18268,1.);
#5510=VECTOR('',#18271,1.);
#5511=VECTOR('',#18276,1.);
#5512=VECTOR('',#18277,1.);
#5513=VECTOR('',#18278,1.);
#5514=VECTOR('',#18281,1.);
#5515=VECTOR('',#18282,1.);
#5516=VECTOR('',#18285,1.);
#5517=VECTOR('',#18286,1.);
#5518=VECTOR('',#18289,1.);
#5519=VECTOR('',#18294,1.);
#5520=VECTOR('',#18295,1.);
#5521=VECTOR('',#18296,1.);
#5522=VECTOR('',#18299,1.);
#5523=VECTOR('',#18300,1.);
#5524=VECTOR('',#18303,1.);
#5525=VECTOR('',#18304,1.);
#5526=VECTOR('',#18307,1.);
#5527=VECTOR('',#18312,1.);
#5528=VECTOR('',#18313,1.);
#5529=VECTOR('',#18314,1.);
#5530=VECTOR('',#18317,1.);
#5531=VECTOR('',#18318,1.);
#5532=VECTOR('',#18321,1.);
#5533=VECTOR('',#18322,1.);
#5534=VECTOR('',#18325,1.);
#5535=VECTOR('',#18330,1.);
#5536=VECTOR('',#18331,1.);
#5537=VECTOR('',#18332,1.);
#5538=VECTOR('',#18335,1.);
#5539=VECTOR('',#18336,1.);
#5540=VECTOR('',#18339,1.);
#5541=VECTOR('',#18340,1.);
#5542=VECTOR('',#18343,1.);
#5543=VECTOR('',#18348,1.);
#5544=VECTOR('',#18349,1.);
#5545=VECTOR('',#18350,1.);
#5546=VECTOR('',#18353,1.);
#5547=VECTOR('',#18354,1.);
#5548=VECTOR('',#18357,1.);
#5549=VECTOR('',#18358,1.);
#5550=VECTOR('',#18361,1.);
#5551=VECTOR('',#18366,2.6);
#5552=VECTOR('',#18375,2.75);
#5553=VECTOR('',#18384,2.6);
#5554=VECTOR('',#18393,2.3);
#5555=VECTOR('',#18394,2.3);
#5556=VECTOR('',#18403,2.6);
#5557=VECTOR('',#18412,2.75);
#5558=VECTOR('',#18421,2.6);
#5559=VECTOR('',#18424,5.3);
#5560=VECTOR('',#18433,3.75);
#5561=VECTOR('',#18442,3.1);
#5562=VECTOR('',#18447,3.155);
#6001=VERTEX_POINT('',#21061);
#6002=VERTEX_POINT('',#21062);
#6003=VERTEX_POINT('',#21064);
#6004=VERTEX_POINT('',#21066);
#6005=VERTEX_POINT('',#21070);
#6006=VERTEX_POINT('',#21072);
#6007=VERTEX_POINT('',#21076);
#6008=VERTEX_POINT('',#21078);
#6009=VERTEX_POINT('',#21086);
#6010=VERTEX_POINT('',#21087);
#6011=VERTEX_POINT('',#21089);
#6012=VERTEX_POINT('',#21091);
#6013=VERTEX_POINT('',#21095);
#6014=VERTEX_POINT('',#21097);
#6015=VERTEX_POINT('',#21099);
#6016=VERTEX_POINT('',#21101);
#6017=VERTEX_POINT('',#21105);
#6018=VERTEX_POINT('',#21109);
#6019=VERTEX_POINT('',#21113);
#6020=VERTEX_POINT('',#21117);
#6021=VERTEX_POINT('',#21118);
#6022=VERTEX_POINT('',#21120);
#6023=VERTEX_POINT('',#21122);
#6024=VERTEX_POINT('',#21126);
#6025=VERTEX_POINT('',#21128);
#6026=VERTEX_POINT('',#21132);
#6027=VERTEX_POINT('',#21134);
#6028=VERTEX_POINT('',#21142);
#6029=VERTEX_POINT('',#21143);
#6030=VERTEX_POINT('',#21145);
#6031=VERTEX_POINT('',#21147);
#6032=VERTEX_POINT('',#21151);
#6033=VERTEX_POINT('',#21153);
#6034=VERTEX_POINT('',#21157);
#6035=VERTEX_POINT('',#21159);
#6036=VERTEX_POINT('',#21167);
#6037=VERTEX_POINT('',#21168);
#6038=VERTEX_POINT('',#21170);
#6039=VERTEX_POINT('',#21172);
#6040=VERTEX_POINT('',#21176);
#6041=VERTEX_POINT('',#21178);
#6042=VERTEX_POINT('',#21182);
#6043=VERTEX_POINT('',#21184);
#6044=VERTEX_POINT('',#21192);
#6045=VERTEX_POINT('',#21193);
#6046=VERTEX_POINT('',#21195);
#6047=VERTEX_POINT('',#21197);
#6048=VERTEX_POINT('',#21201);
#6049=VERTEX_POINT('',#21202);
#6050=VERTEX_POINT('',#21204);
#6051=VERTEX_POINT('',#21206);
#6052=VERTEX_POINT('',#21210);
#6053=VERTEX_POINT('',#21212);
#6054=VERTEX_POINT('',#21219);
#6055=VERTEX_POINT('',#21223);
#6056=VERTEX_POINT('',#21225);
#6057=VERTEX_POINT('',#21227);
#6058=VERTEX_POINT('',#21231);
#6059=VERTEX_POINT('',#21233);
#6060=VERTEX_POINT('',#21237);
#6061=VERTEX_POINT('',#21239);
#6062=VERTEX_POINT('',#21241);
#6063=VERTEX_POINT('',#21243);
#6064=VERTEX_POINT('',#21245);
#6065=VERTEX_POINT('',#21248);
#6066=VERTEX_POINT('',#21250);
#6067=VERTEX_POINT('',#21252);
#6068=VERTEX_POINT('',#21255);
#6069=VERTEX_POINT('',#21258);
#6070=VERTEX_POINT('',#21259);
#6071=VERTEX_POINT('',#21261);
#6072=VERTEX_POINT('',#21263);
#6073=VERTEX_POINT('',#21267);
#6074=VERTEX_POINT('',#21269);
#6075=VERTEX_POINT('',#21273);
#6076=VERTEX_POINT('',#21275);
#6077=VERTEX_POINT('',#21283);
#6078=VERTEX_POINT('',#21284);
#6079=VERTEX_POINT('',#21286);
#6080=VERTEX_POINT('',#21288);
#6081=VERTEX_POINT('',#21292);
#6082=VERTEX_POINT('',#21293);
#6083=VERTEX_POINT('',#21295);
#6084=VERTEX_POINT('',#21297);
#6085=VERTEX_POINT('',#21304);
#6086=VERTEX_POINT('',#21305);
#6087=VERTEX_POINT('',#21310);
#6088=VERTEX_POINT('',#21314);
#6089=VERTEX_POINT('',#21315);
#6090=VERTEX_POINT('',#21317);
#6091=VERTEX_POINT('',#21319);
#6092=VERTEX_POINT('',#21323);
#6093=VERTEX_POINT('',#21325);
#6094=VERTEX_POINT('',#21329);
#6095=VERTEX_POINT('',#21331);
#6096=VERTEX_POINT('',#21339);
#6097=VERTEX_POINT('',#21340);
#6098=VERTEX_POINT('',#21342);
#6099=VERTEX_POINT('',#21344);
#6100=VERTEX_POINT('',#21348);
#6101=VERTEX_POINT('',#21350);
#6102=VERTEX_POINT('',#21354);
#6103=VERTEX_POINT('',#21356);
#6104=VERTEX_POINT('',#21364);
#6105=VERTEX_POINT('',#21365);
#6106=VERTEX_POINT('',#21367);
#6107=VERTEX_POINT('',#21369);
#6108=VERTEX_POINT('',#21373);
#6109=VERTEX_POINT('',#21375);
#6110=VERTEX_POINT('',#21379);
#6111=VERTEX_POINT('',#21381);
#6112=VERTEX_POINT('',#21389);
#6113=VERTEX_POINT('',#21390);
#6114=VERTEX_POINT('',#21392);
#6115=VERTEX_POINT('',#21394);
#6116=VERTEX_POINT('',#21398);
#6117=VERTEX_POINT('',#21400);
#6118=VERTEX_POINT('',#21404);
#6119=VERTEX_POINT('',#21405);
#6120=VERTEX_POINT('',#21407);
#6121=VERTEX_POINT('',#21409);
#6122=VERTEX_POINT('',#21416);
#6123=VERTEX_POINT('',#21420);
#6124=VERTEX_POINT('',#21422);
#6125=VERTEX_POINT('',#21424);
#6126=VERTEX_POINT('',#21428);
#6127=VERTEX_POINT('',#21430);
#6128=VERTEX_POINT('',#21432);
#6129=VERTEX_POINT('',#21436);
#6130=VERTEX_POINT('',#21438);
#6131=VERTEX_POINT('',#21440);
#6132=VERTEX_POINT('',#21442);
#6133=VERTEX_POINT('',#21444);
#6134=VERTEX_POINT('',#21446);
#6135=VERTEX_POINT('',#21448);
#6136=VERTEX_POINT('',#21450);
#6137=VERTEX_POINT('',#21452);
#6138=VERTEX_POINT('',#21455);
#6139=VERTEX_POINT('',#21457);
#6140=VERTEX_POINT('',#21459);
#6141=VERTEX_POINT('',#21461);
#6142=VERTEX_POINT('',#21463);
#6143=VERTEX_POINT('',#21466);
#6144=VERTEX_POINT('',#21468);
#6145=VERTEX_POINT('',#21470);
#6146=VERTEX_POINT('',#21473);
#6147=VERTEX_POINT('',#21474);
#6148=VERTEX_POINT('',#21476);
#6149=VERTEX_POINT('',#21478);
#6150=VERTEX_POINT('',#21482);
#6151=VERTEX_POINT('',#21484);
#6152=VERTEX_POINT('',#21488);
#6153=VERTEX_POINT('',#21490);
#6154=VERTEX_POINT('',#21494);
#6155=VERTEX_POINT('',#21496);
#6156=VERTEX_POINT('',#21500);
#6157=VERTEX_POINT('',#21502);
#6158=VERTEX_POINT('',#21510);
#6159=VERTEX_POINT('',#21511);
#6160=VERTEX_POINT('',#21513);
#6161=VERTEX_POINT('',#21515);
#6162=VERTEX_POINT('',#21519);
#6163=VERTEX_POINT('',#21521);
#6164=VERTEX_POINT('',#21525);
#6165=VERTEX_POINT('',#21527);
#6166=VERTEX_POINT('',#21531);
#6167=VERTEX_POINT('',#21533);
#6168=VERTEX_POINT('',#21537);
#6169=VERTEX_POINT('',#21539);
#6170=VERTEX_POINT('',#21541);
#6171=VERTEX_POINT('',#21544);
#6172=VERTEX_POINT('',#21546);
#6173=VERTEX_POINT('',#21549);
#6174=VERTEX_POINT('',#21551);
#6175=VERTEX_POINT('',#21553);
#6176=VERTEX_POINT('',#21555);
#6177=VERTEX_POINT('',#21559);
#6178=VERTEX_POINT('',#21560);
#6179=VERTEX_POINT('',#21562);
#6180=VERTEX_POINT('',#21567);
#6181=VERTEX_POINT('',#21574);
#6182=VERTEX_POINT('',#21576);
#6183=VERTEX_POINT('',#21580);
#6184=VERTEX_POINT('',#21582);
#6185=VERTEX_POINT('',#21586);
#6186=VERTEX_POINT('',#21588);
#6187=VERTEX_POINT('',#21595);
#6188=VERTEX_POINT('',#21597);
#6189=VERTEX_POINT('',#21604);
#6190=VERTEX_POINT('',#21606);
#6191=VERTEX_POINT('',#21610);
#6192=VERTEX_POINT('',#21612);
#6193=VERTEX_POINT('',#21616);
#6194=VERTEX_POINT('',#21618);
#6195=VERTEX_POINT('',#21625);
#6196=VERTEX_POINT('',#21627);
#6197=VERTEX_POINT('',#21634);
#6198=VERTEX_POINT('',#21636);
#6199=VERTEX_POINT('',#21643);
#6200=VERTEX_POINT('',#21645);
#6201=VERTEX_POINT('',#21668);
#6202=VERTEX_POINT('',#21670);
#6203=VERTEX_POINT('',#21672);
#6204=VERTEX_POINT('',#21674);
#6205=VERTEX_POINT('',#21676);
#6206=VERTEX_POINT('',#21679);
#6207=VERTEX_POINT('',#21680);
#6208=VERTEX_POINT('',#21717);
#6209=VERTEX_POINT('',#21721);
#6210=VERTEX_POINT('',#21725);
#6211=VERTEX_POINT('',#21726);
#6212=VERTEX_POINT('',#21730);
#6213=VERTEX_POINT('',#21732);
#6214=VERTEX_POINT('',#21747);
#6215=VERTEX_POINT('',#21762);
#6216=VERTEX_POINT('',#21793);
#6217=VERTEX_POINT('',#21795);
#6218=VERTEX_POINT('',#21797);
#6219=VERTEX_POINT('',#21810);
#6220=VERTEX_POINT('',#21812);
#6221=VERTEX_POINT('',#21814);
#6222=VERTEX_POINT('',#21816);
#6223=VERTEX_POINT('',#21818);
#6224=VERTEX_POINT('',#21820);
#6225=VERTEX_POINT('',#21822);
#6226=VERTEX_POINT('',#21824);
#6227=VERTEX_POINT('',#21827);
#6228=VERTEX_POINT('',#21829);
#6229=VERTEX_POINT('',#21831);
#6230=VERTEX_POINT('',#21834);
#6231=VERTEX_POINT('',#21835);
#6232=VERTEX_POINT('',#21837);
#6233=VERTEX_POINT('',#21839);
#6234=VERTEX_POINT('',#21842);
#6235=VERTEX_POINT('',#21843);
#6236=VERTEX_POINT('',#21845);
#6237=VERTEX_POINT('',#21847);
#6238=VERTEX_POINT('',#21850);
#6239=VERTEX_POINT('',#21851);
#6240=VERTEX_POINT('',#21853);
#6241=VERTEX_POINT('',#21855);
#6242=VERTEX_POINT('',#21858);
#6243=VERTEX_POINT('',#21859);
#6244=VERTEX_POINT('',#21861);
#6245=VERTEX_POINT('',#21863);
#6246=VERTEX_POINT('',#21866);
#6247=VERTEX_POINT('',#21867);
#6248=VERTEX_POINT('',#21869);
#6249=VERTEX_POINT('',#21871);
#6250=VERTEX_POINT('',#21874);
#6251=VERTEX_POINT('',#21875);
#6252=VERTEX_POINT('',#21877);
#6253=VERTEX_POINT('',#21879);
#6254=VERTEX_POINT('',#21883);
#6255=VERTEX_POINT('',#21884);
#6256=VERTEX_POINT('',#21888);
#6257=VERTEX_POINT('',#21891);
#6258=VERTEX_POINT('',#21892);
#6259=VERTEX_POINT('',#22006);
#6260=VERTEX_POINT('',#22007);
#6261=VERTEX_POINT('',#22011);
#6262=VERTEX_POINT('',#22039);
#6263=VERTEX_POINT('',#22040);
#6264=VERTEX_POINT('',#22044);
#6265=VERTEX_POINT('',#22050);
#6266=VERTEX_POINT('',#22051);
#6267=VERTEX_POINT('',#22055);
#6268=VERTEX_POINT('',#22061);
#6269=VERTEX_POINT('',#22062);
#6270=VERTEX_POINT('',#22066);
#6271=VERTEX_POINT('',#22070);
#6272=VERTEX_POINT('',#22074);
#6273=VERTEX_POINT('',#22075);
#6274=VERTEX_POINT('',#22079);
#6275=VERTEX_POINT('',#22085);
#6276=VERTEX_POINT('',#22086);
#6277=VERTEX_POINT('',#22090);
#6278=VERTEX_POINT('',#22094);
#6279=VERTEX_POINT('',#22098);
#6280=VERTEX_POINT('',#22099);
#6281=VERTEX_POINT('',#22103);
#6282=VERTEX_POINT('',#22109);
#6283=VERTEX_POINT('',#22110);
#6284=VERTEX_POINT('',#22114);
#6285=VERTEX_POINT('',#22118);
#6286=VERTEX_POINT('',#22122);
#6287=VERTEX_POINT('',#22123);
#6288=VERTEX_POINT('',#22127);
#6289=VERTEX_POINT('',#22133);
#6290=VERTEX_POINT('',#22134);
#6291=VERTEX_POINT('',#22138);
#6292=VERTEX_POINT('',#22142);
#6293=VERTEX_POINT('',#22146);
#6294=VERTEX_POINT('',#22147);
#6295=VERTEX_POINT('',#22151);
#6296=VERTEX_POINT('',#22157);
#6297=VERTEX_POINT('',#22158);
#6298=VERTEX_POINT('',#22162);
#6299=VERTEX_POINT('',#22168);
#6300=VERTEX_POINT('',#22169);
#6301=VERTEX_POINT('',#22173);
#6302=VERTEX_POINT('',#22179);
#6303=VERTEX_POINT('',#22180);
#6304=VERTEX_POINT('',#22185);
#6305=VERTEX_POINT('',#22191);
#6306=VERTEX_POINT('',#22193);
#6307=VERTEX_POINT('',#22197);
#6308=VERTEX_POINT('',#22201);
#6309=VERTEX_POINT('',#22203);
#6310=VERTEX_POINT('',#22207);
#6311=VERTEX_POINT('',#22211);
#6312=VERTEX_POINT('',#22213);
#6313=VERTEX_POINT('',#22217);
#6314=VERTEX_POINT('',#22221);
#6315=VERTEX_POINT('',#22223);
#6316=VERTEX_POINT('',#22227);
#6317=VERTEX_POINT('',#22231);
#6318=VERTEX_POINT('',#22237);
#6319=VERTEX_POINT('',#22241);
#6320=VERTEX_POINT('',#22247);
#6321=VERTEX_POINT('',#22249);
#6322=VERTEX_POINT('',#22251);
#6323=VERTEX_POINT('',#22253);
#6324=VERTEX_POINT('',#22255);
#6325=VERTEX_POINT('',#22257);
#6326=VERTEX_POINT('',#22260);
#6327=VERTEX_POINT('',#22263);
#6328=VERTEX_POINT('',#22265);
#6329=VERTEX_POINT('',#22269);
#6330=VERTEX_POINT('',#22274);
#6331=VERTEX_POINT('',#22279);
#6332=VERTEX_POINT('',#22281);
#6333=VERTEX_POINT('',#22283);
#6334=VERTEX_POINT('',#22292);
#6335=VERTEX_POINT('',#22297);
#6336=VERTEX_POINT('',#22301);
#6337=VERTEX_POINT('',#22303);
#6338=VERTEX_POINT('',#22305);
#6339=VERTEX_POINT('',#22307);
#6340=VERTEX_POINT('',#22309);
#6341=VERTEX_POINT('',#22311);
#6342=VERTEX_POINT('',#22327);
#6343=VERTEX_POINT('',#22329);
#6344=VERTEX_POINT('',#22333);
#6345=VERTEX_POINT('',#22337);
#6346=VERTEX_POINT('',#22344);
#6347=VERTEX_POINT('',#22346);
#6348=VERTEX_POINT('',#22350);
#6349=VERTEX_POINT('',#22354);
#6350=VERTEX_POINT('',#22361);
#6351=VERTEX_POINT('',#22363);
#6352=VERTEX_POINT('',#22367);
#6353=VERTEX_POINT('',#22371);
#6354=VERTEX_POINT('',#22378);
#6355=VERTEX_POINT('',#22380);
#6356=VERTEX_POINT('',#22384);
#6357=VERTEX_POINT('',#22388);
#6358=VERTEX_POINT('',#22395);
#6359=VERTEX_POINT('',#22397);
#6360=VERTEX_POINT('',#22401);
#6361=VERTEX_POINT('',#22405);
#6362=VERTEX_POINT('',#22412);
#6363=VERTEX_POINT('',#22414);
#6364=VERTEX_POINT('',#22418);
#6365=VERTEX_POINT('',#22422);
#6366=VERTEX_POINT('',#22429);
#6367=VERTEX_POINT('',#22433);
#6368=VERTEX_POINT('',#22436);
#6369=VERTEX_POINT('',#22440);
#6370=VERTEX_POINT('',#22443);
#6371=VERTEX_POINT('',#22447);
#6372=VERTEX_POINT('',#22450);
#6373=VERTEX_POINT('',#22452);
#6374=VERTEX_POINT('',#22471);
#6375=VERTEX_POINT('',#22490);
#6376=VERTEX_POINT('',#22529);
#6377=VERTEX_POINT('',#22532);
#6378=VERTEX_POINT('',#22536);
#6379=VERTEX_POINT('',#22539);
#6380=VERTEX_POINT('',#22543);
#6381=VERTEX_POINT('',#22548);
#6382=VERTEX_POINT('',#22552);
#6383=VERTEX_POINT('',#22555);
#6384=VERTEX_POINT('',#22559);
#6385=VERTEX_POINT('',#22562);
#7547=EDGE_CURVE('',#6001,#6002,#4281,.T.);
#7548=EDGE_CURVE('',#6001,#6003,#4282,.T.);
#7549=EDGE_CURVE('',#6003,#6004,#4283,.T.);
#7550=EDGE_CURVE('',#6002,#6004,#4284,.T.);
#7551=EDGE_CURVE('',#6005,#6001,#4285,.T.);
#7552=EDGE_CURVE('',#6005,#6006,#4286,.T.);
#7553=EDGE_CURVE('',#6006,#6003,#4287,.T.);
#7554=EDGE_CURVE('',#6007,#6005,#4288,.T.);
#7555=EDGE_CURVE('',#6007,#6008,#4289,.T.);
#7556=EDGE_CURVE('',#6008,#6006,#4290,.T.);
#7557=EDGE_CURVE('',#6002,#6007,#4291,.T.);
#7558=EDGE_CURVE('',#6004,#6008,#4292,.T.);
#7559=EDGE_CURVE('',#6009,#6010,#4293,.T.);
#7560=EDGE_CURVE('',#6011,#6009,#4294,.T.);
#7561=EDGE_CURVE('',#6011,#6012,#4295,.T.);
#7562=EDGE_CURVE('',#6012,#6010,#4296,.T.);
#7563=EDGE_CURVE('',#6010,#6013,#4297,.T.);
#7564=EDGE_CURVE('',#6014,#6012,#4298,.T.);
#7565=EDGE_CURVE('',#6015,#6014,#4299,.T.);
#7566=EDGE_CURVE('',#6016,#6015,#4300,.T.);
#7567=EDGE_CURVE('',#6013,#6016,#4301,.T.);
#7568=EDGE_CURVE('',#6017,#6011,#4302,.T.);
#7569=EDGE_CURVE('',#6017,#6014,#4303,.T.);
#7570=EDGE_CURVE('',#6018,#6017,#4304,.T.);
#7571=EDGE_CURVE('',#6018,#6015,#4305,.T.);
#7572=EDGE_CURVE('',#6016,#6019,#4306,.T.);
#7573=EDGE_CURVE('',#6019,#6018,#4307,.T.);
#7574=EDGE_CURVE('',#6020,#6021,#4308,.T.);
#7575=EDGE_CURVE('',#6020,#6022,#4309,.T.);
#7576=EDGE_CURVE('',#6022,#6023,#4310,.T.);
#7577=EDGE_CURVE('',#6021,#6023,#4311,.T.);
#7578=EDGE_CURVE('',#6024,#6020,#4312,.T.);
#7579=EDGE_CURVE('',#6024,#6025,#4313,.T.);
#7580=EDGE_CURVE('',#6025,#6022,#4314,.T.);
#7581=EDGE_CURVE('',#6026,#6024,#4315,.T.);
#7582=EDGE_CURVE('',#6026,#6027,#4316,.T.);
#7583=EDGE_CURVE('',#6027,#6025,#4317,.T.);
#7584=EDGE_CURVE('',#6021,#6026,#4318,.T.);
#7585=EDGE_CURVE('',#6023,#6027,#4319,.T.);
#7586=EDGE_CURVE('',#6028,#6029,#4320,.T.);
#7587=EDGE_CURVE('',#6028,#6030,#4321,.T.);
#7588=EDGE_CURVE('',#6030,#6031,#4322,.T.);
#7589=EDGE_CURVE('',#6029,#6031,#4323,.T.);
#7590=EDGE_CURVE('',#6032,#6028,#4324,.T.);
#7591=EDGE_CURVE('',#6032,#6033,#4325,.T.);
#7592=EDGE_CURVE('',#6033,#6030,#4326,.T.);
#7593=EDGE_CURVE('',#6034,#6032,#4327,.T.);
#7594=EDGE_CURVE('',#6034,#6035,#4328,.T.);
#7595=EDGE_CURVE('',#6035,#6033,#4329,.T.);
#7596=EDGE_CURVE('',#6029,#6034,#4330,.T.);
#7597=EDGE_CURVE('',#6031,#6035,#4331,.T.);
#7598=EDGE_CURVE('',#6036,#6037,#4332,.T.);
#7599=EDGE_CURVE('',#6036,#6038,#4333,.T.);
#7600=EDGE_CURVE('',#6038,#6039,#4334,.T.);
#7601=EDGE_CURVE('',#6037,#6039,#4335,.T.);
#7602=EDGE_CURVE('',#6040,#6036,#4336,.T.);
#7603=EDGE_CURVE('',#6040,#6041,#4337,.T.);
#7604=EDGE_CURVE('',#6041,#6038,#4338,.T.);
#7605=EDGE_CURVE('',#6042,#6040,#4339,.T.);
#7606=EDGE_CURVE('',#6042,#6043,#4340,.T.);
#7607=EDGE_CURVE('',#6043,#6041,#4341,.T.);
#7608=EDGE_CURVE('',#6037,#6042,#4342,.T.);
#7609=EDGE_CURVE('',#6039,#6043,#4343,.T.);
#7610=EDGE_CURVE('',#6044,#6045,#4344,.T.);
#7611=EDGE_CURVE('',#6044,#6046,#4345,.T.);
#7612=EDGE_CURVE('',#6047,#6046,#4346,.T.);
#7613=EDGE_CURVE('',#6045,#6047,#4347,.T.);
#7614=EDGE_CURVE('',#6048,#6049,#4348,.T.);
#7615=EDGE_CURVE('',#6050,#6048,#4349,.T.);
#7616=EDGE_CURVE('',#6050,#6051,#4350,.T.);
#7617=EDGE_CURVE('',#6051,#6049,#4351,.T.);
#7618=EDGE_CURVE('',#6052,#6050,#4352,.T.);
#7619=EDGE_CURVE('',#6052,#6053,#4353,.T.);
#7620=EDGE_CURVE('',#6053,#6051,#4354,.T.);
#7621=EDGE_CURVE('',#6047,#6052,#4355,.T.);
#7622=EDGE_CURVE('',#6046,#6053,#4356,.T.);
#7623=EDGE_CURVE('',#6054,#6044,#4357,.T.);
#7624=EDGE_CURVE('',#6049,#6054,#4358,.T.);
#7625=EDGE_CURVE('',#6013,#6055,#4359,.T.);
#7626=EDGE_CURVE('',#6055,#6056,#4360,.T.);
#7627=EDGE_CURVE('',#6056,#6057,#4361,.T.);
#7628=EDGE_CURVE('',#6009,#6057,#4362,.T.);
#7629=EDGE_CURVE('',#6058,#6019,#4363,.T.);
#7630=EDGE_CURVE('',#6059,#6058,#4364,.T.);
#7631=EDGE_CURVE('',#6055,#6059,#4365,.T.);
#7632=EDGE_CURVE('',#6057,#6060,#4366,.T.);
#7633=EDGE_CURVE('',#6061,#6060,#4367,.T.);
#7634=EDGE_CURVE('',#6062,#6061,#4368,.T.);
#7635=EDGE_CURVE('',#6063,#6062,#4369,.T.);
#7636=EDGE_CURVE('',#6063,#6064,#4370,.T.);
#7637=EDGE_CURVE('',#6064,#6045,#4371,.T.);
#7638=EDGE_CURVE('',#6048,#6065,#4372,.T.);
#7639=EDGE_CURVE('',#6066,#6065,#4373,.T.);
#7640=EDGE_CURVE('',#6067,#6066,#4374,.T.);
#7641=EDGE_CURVE('',#6058,#6067,#4375,.T.);
#7642=EDGE_CURVE('',#6068,#6068,#1754,.T.);
#7643=EDGE_CURVE('',#6069,#6070,#4376,.T.);
#7644=EDGE_CURVE('',#6069,#6071,#4377,.T.);
#7645=EDGE_CURVE('',#6071,#6072,#4378,.T.);
#7646=EDGE_CURVE('',#6070,#6072,#4379,.T.);
#7647=EDGE_CURVE('',#6073,#6069,#4380,.T.);
#7648=EDGE_CURVE('',#6073,#6074,#4381,.T.);
#7649=EDGE_CURVE('',#6074,#6071,#4382,.T.);
#7650=EDGE_CURVE('',#6075,#6073,#4383,.T.);
#7651=EDGE_CURVE('',#6075,#6076,#4384,.T.);
#7652=EDGE_CURVE('',#6076,#6074,#4385,.T.);
#7653=EDGE_CURVE('',#6070,#6075,#4386,.T.);
#7654=EDGE_CURVE('',#6072,#6076,#4387,.T.);
#7655=EDGE_CURVE('',#6077,#6078,#4388,.T.);
#7656=EDGE_CURVE('',#6077,#6079,#4389,.T.);
#7657=EDGE_CURVE('',#6080,#6079,#4390,.T.);
#7658=EDGE_CURVE('',#6078,#6080,#4391,.T.);
#7659=EDGE_CURVE('',#6081,#6082,#4392,.T.);
#7660=EDGE_CURVE('',#6081,#6083,#4393,.T.);
#7661=EDGE_CURVE('',#6083,#6084,#4394,.T.);
#7662=EDGE_CURVE('',#6082,#6084,#4395,.T.);
#7663=EDGE_CURVE('',#6080,#6081,#4396,.T.);
#7664=EDGE_CURVE('',#6079,#6083,#4397,.T.);
#7665=EDGE_CURVE('',#6085,#6086,#4398,.T.);
#7666=EDGE_CURVE('',#6082,#6085,#4399,.T.);
#7667=EDGE_CURVE('',#6084,#6086,#4400,.T.);
#7668=EDGE_CURVE('',#6087,#6077,#4401,.T.);
#7669=EDGE_CURVE('',#6086,#6087,#4402,.T.);
#7670=EDGE_CURVE('',#6088,#6089,#4403,.T.);
#7671=EDGE_CURVE('',#6088,#6090,#4404,.T.);
#7672=EDGE_CURVE('',#6090,#6091,#4405,.T.);
#7673=EDGE_CURVE('',#6089,#6091,#4406,.T.);
#7674=EDGE_CURVE('',#6092,#6088,#4407,.T.);
#7675=EDGE_CURVE('',#6092,#6093,#4408,.T.);
#7676=EDGE_CURVE('',#6093,#6090,#4409,.T.);
#7677=EDGE_CURVE('',#6094,#6092,#4410,.T.);
#7678=EDGE_CURVE('',#6094,#6095,#4411,.T.);
#7679=EDGE_CURVE('',#6095,#6093,#4412,.T.);
#7680=EDGE_CURVE('',#6089,#6094,#4413,.T.);
#7681=EDGE_CURVE('',#6091,#6095,#4414,.T.);
#7682=EDGE_CURVE('',#6096,#6097,#4415,.T.);
#7683=EDGE_CURVE('',#6096,#6098,#4416,.T.);
#7684=EDGE_CURVE('',#6098,#6099,#4417,.T.);
#7685=EDGE_CURVE('',#6097,#6099,#4418,.T.);
#7686=EDGE_CURVE('',#6100,#6096,#4419,.T.);
#7687=EDGE_CURVE('',#6100,#6101,#4420,.T.);
#7688=EDGE_CURVE('',#6101,#6098,#4421,.T.);
#7689=EDGE_CURVE('',#6102,#6100,#4422,.T.);
#7690=EDGE_CURVE('',#6102,#6103,#4423,.T.);
#7691=EDGE_CURVE('',#6103,#6101,#4424,.T.);
#7692=EDGE_CURVE('',#6097,#6102,#4425,.T.);
#7693=EDGE_CURVE('',#6099,#6103,#4426,.T.);
#7694=EDGE_CURVE('',#6104,#6105,#4427,.T.);
#7695=EDGE_CURVE('',#6104,#6106,#4428,.T.);
#7696=EDGE_CURVE('',#6106,#6107,#4429,.T.);
#7697=EDGE_CURVE('',#6105,#6107,#4430,.T.);
#7698=EDGE_CURVE('',#6108,#6104,#4431,.T.);
#7699=EDGE_CURVE('',#6108,#6109,#4432,.T.);
#7700=EDGE_CURVE('',#6109,#6106,#4433,.T.);
#7701=EDGE_CURVE('',#6110,#6108,#4434,.T.);
#7702=EDGE_CURVE('',#6110,#6111,#4435,.T.);
#7703=EDGE_CURVE('',#6111,#6109,#4436,.T.);
#7704=EDGE_CURVE('',#6105,#6110,#4437,.T.);
#7705=EDGE_CURVE('',#6107,#6111,#4438,.T.);
#7706=EDGE_CURVE('',#6112,#6113,#4439,.T.);
#7707=EDGE_CURVE('',#6112,#6114,#4440,.T.);
#7708=EDGE_CURVE('',#6115,#6114,#4441,.T.);
#7709=EDGE_CURVE('',#6113,#6115,#4442,.T.);
#7710=EDGE_CURVE('',#6115,#6116,#4443,.T.);
#7711=EDGE_CURVE('',#6114,#6117,#4444,.T.);
#7712=EDGE_CURVE('',#6116,#6117,#4445,.T.);
#7713=EDGE_CURVE('',#6118,#6119,#4446,.T.);
#7714=EDGE_CURVE('',#6120,#6118,#4447,.T.);
#7715=EDGE_CURVE('',#6120,#6121,#4448,.T.);
#7716=EDGE_CURVE('',#6121,#6119,#4449,.T.);
#7717=EDGE_CURVE('',#6116,#6120,#4450,.T.);
#7718=EDGE_CURVE('',#6117,#6121,#4451,.T.);
#7719=EDGE_CURVE('',#6122,#6112,#4452,.T.);
#7720=EDGE_CURVE('',#6119,#6122,#4453,.T.);
#7721=EDGE_CURVE('',#6123,#6078,#4454,.T.);
#7722=EDGE_CURVE('',#6123,#6124,#4455,.T.);
#7723=EDGE_CURVE('',#6124,#6125,#4456,.T.);
#7724=EDGE_CURVE('',#6125,#6087,#4457,.T.);
#7725=EDGE_CURVE('',#6126,#6113,#4458,.T.);
#7726=EDGE_CURVE('',#6127,#6126,#4459,.T.);
#7727=EDGE_CURVE('',#6128,#6127,#4460,.T.);
#7728=EDGE_CURVE('',#6128,#6122,#4461,.T.);
#7729=EDGE_CURVE('',#6085,#6129,#4462,.T.);
#7730=EDGE_CURVE('',#6130,#6129,#4463,.T.);
#7731=EDGE_CURVE('',#6131,#6130,#4464,.T.);
#7732=EDGE_CURVE('',#6131,#6132,#1755,.T.);
#7733=EDGE_CURVE('',#6132,#6133,#1756,.T.);
#7734=EDGE_CURVE('',#6134,#6133,#4465,.T.);
#7735=EDGE_CURVE('',#6134,#6135,#1757,.T.);
#7736=EDGE_CURVE('',#6135,#6136,#1758,.T.);
#7737=EDGE_CURVE('',#6137,#6136,#4466,.T.);
#7738=EDGE_CURVE('',#6126,#6137,#4467,.T.);
#7739=EDGE_CURVE('',#6118,#6138,#4468,.T.);
#7740=EDGE_CURVE('',#6138,#6139,#4469,.T.);
#7741=EDGE_CURVE('',#6140,#6139,#4470,.T.);
#7742=EDGE_CURVE('',#6141,#6140,#4471,.T.);
#7743=EDGE_CURVE('',#6142,#6141,#4472,.T.);
#7744=EDGE_CURVE('',#6142,#6123,#4473,.T.);
#7745=EDGE_CURVE('',#6143,#6143,#1759,.T.);
#7746=EDGE_CURVE('',#6144,#6144,#1760,.T.);
#7747=EDGE_CURVE('',#6145,#6145,#1761,.T.);
#7748=EDGE_CURVE('',#6146,#6147,#1762,.T.);
#7749=EDGE_CURVE('',#6146,#6148,#4474,.T.);
#7750=EDGE_CURVE('',#6148,#6149,#1763,.T.);
#7751=EDGE_CURVE('',#6147,#6149,#4475,.T.);
#7752=EDGE_CURVE('',#6150,#6146,#1764,.T.);
#7753=EDGE_CURVE('',#6150,#6151,#4476,.T.);
#7754=EDGE_CURVE('',#6151,#6148,#1765,.T.);
#7755=EDGE_CURVE('',#6152,#6150,#4477,.T.);
#7756=EDGE_CURVE('',#6152,#6153,#4478,.T.);
#7757=EDGE_CURVE('',#6153,#6151,#4479,.T.);
#7758=EDGE_CURVE('',#6154,#6152,#4480,.T.);
#7759=EDGE_CURVE('',#6154,#6155,#4481,.T.);
#7760=EDGE_CURVE('',#6155,#6153,#4482,.T.);
#7761=EDGE_CURVE('',#6156,#6154,#4483,.T.);
#7762=EDGE_CURVE('',#6156,#6157,#4484,.T.);
#7763=EDGE_CURVE('',#6157,#6155,#4485,.T.);
#7764=EDGE_CURVE('',#6147,#6156,#1766,.T.);
#7765=EDGE_CURVE('',#6149,#6157,#1767,.T.);
#7766=EDGE_CURVE('',#6158,#6159,#4486,.T.);
#7767=EDGE_CURVE('',#6158,#6160,#4487,.T.);
#7768=EDGE_CURVE('',#6160,#6161,#4488,.T.);
#7769=EDGE_CURVE('',#6159,#6161,#4489,.T.);
#7770=EDGE_CURVE('',#6162,#6158,#4490,.T.);
#7771=EDGE_CURVE('',#6162,#6163,#4491,.T.);
#7772=EDGE_CURVE('',#6163,#6160,#4492,.T.);
#7773=EDGE_CURVE('',#6164,#6162,#4493,.T.);
#7774=EDGE_CURVE('',#6164,#6165,#4494,.T.);
#7775=EDGE_CURVE('',#6165,#6163,#4495,.T.);
#7776=EDGE_CURVE('',#6161,#6166,#1768,.T.);
#7777=EDGE_CURVE('',#6167,#6165,#1769,.T.);
#7778=EDGE_CURVE('',#6166,#6167,#1770,.T.);
#7779=EDGE_CURVE('',#6159,#6168,#1771,.T.);
#7780=EDGE_CURVE('',#6168,#6169,#1772,.T.);
#7781=EDGE_CURVE('',#6169,#6170,#1773,.T.);
#7782=EDGE_CURVE('',#6170,#6127,#4496,.T.);
#7783=EDGE_CURVE('',#6171,#6137,#1774,.T.);
#7784=EDGE_CURVE('',#6171,#6172,#4497,.T.);
#7785=EDGE_CURVE('',#6066,#6172,#1775,.T.);
#7786=EDGE_CURVE('',#6065,#6173,#4498,.T.);
#7787=EDGE_CURVE('',#6173,#6174,#4499,.T.);
#7788=EDGE_CURVE('',#6174,#6175,#1776,.T.);
#7789=EDGE_CURVE('',#6175,#6176,#1777,.T.);
#7790=EDGE_CURVE('',#6176,#6164,#1778,.T.);
#7791=EDGE_CURVE('',#6177,#6178,#1779,.T.);
#7792=EDGE_CURVE('',#6178,#6179,#363,.T.);
#7793=EDGE_CURVE('',#6179,#6180,#1780,.T.);
#7794=EDGE_CURVE('',#6177,#6180,#364,.T.);
#7795=EDGE_CURVE('',#6178,#6181,#1781,.T.);
#7796=EDGE_CURVE('',#6181,#6182,#359,.T.);
#7797=EDGE_CURVE('',#6182,#6179,#1782,.T.);
#7798=EDGE_CURVE('',#6181,#6183,#4500,.T.);
#7799=EDGE_CURVE('',#6183,#6184,#360,.T.);
#7800=EDGE_CURVE('',#6184,#6182,#4501,.T.);
#7801=EDGE_CURVE('',#6183,#6185,#1783,.T.);
#7802=EDGE_CURVE('',#6185,#6186,#365,.T.);
#7803=EDGE_CURVE('',#6186,#6184,#1784,.T.);
#7804=EDGE_CURVE('',#6185,#6187,#1785,.T.);
#7805=EDGE_CURVE('',#6187,#6188,#366,.T.);
#7806=EDGE_CURVE('',#6188,#6186,#1786,.T.);
#7807=EDGE_CURVE('',#6187,#6189,#1787,.T.);
#7808=EDGE_CURVE('',#6189,#6190,#361,.T.);
#7809=EDGE_CURVE('',#6190,#6188,#1788,.T.);
#7810=EDGE_CURVE('',#6189,#6191,#4502,.T.);
#7811=EDGE_CURVE('',#6191,#6192,#362,.T.);
#7812=EDGE_CURVE('',#6192,#6190,#4503,.T.);
#7813=EDGE_CURVE('',#6193,#6192,#1789,.T.);
#7814=EDGE_CURVE('',#6191,#6194,#1790,.T.);
#7815=EDGE_CURVE('',#6194,#6193,#367,.T.);
#7816=EDGE_CURVE('',#6195,#6193,#1791,.T.);
#7817=EDGE_CURVE('',#6194,#6196,#1792,.T.);
#7818=EDGE_CURVE('',#6196,#6195,#368,.T.);
#7819=EDGE_CURVE('',#6197,#6195,#1793,.T.);
#7820=EDGE_CURVE('',#6196,#6198,#1794,.T.);
#7821=EDGE_CURVE('',#6198,#6197,#369,.T.);
#7822=EDGE_CURVE('',#6199,#6197,#1795,.T.);
#7823=EDGE_CURVE('',#6198,#6200,#1796,.T.);
#7824=EDGE_CURVE('',#6200,#6199,#370,.T.);
#7825=EDGE_CURVE('',#6180,#6199,#1797,.T.);
#7826=EDGE_CURVE('',#6200,#6177,#1798,.T.);
#7827=EDGE_CURVE('',#6175,#6193,#4504,.T.);
#7828=EDGE_CURVE('',#6174,#6192,#4505,.T.);
#7829=EDGE_CURVE('',#6176,#6195,#4506,.T.);
#7830=EDGE_CURVE('',#6197,#6167,#4507,.T.);
#7831=EDGE_CURVE('',#6199,#6166,#4508,.T.);
#7832=EDGE_CURVE('',#6168,#6180,#4509,.T.);
#7833=EDGE_CURVE('',#6169,#6179,#4510,.T.);
#7834=EDGE_CURVE('',#6201,#6201,#1799,.T.);
#7835=EDGE_CURVE('',#6202,#6202,#1800,.T.);
#7836=EDGE_CURVE('',#6203,#6203,#1801,.T.);
#7837=EDGE_CURVE('',#6204,#6204,#1802,.T.);
#7838=EDGE_CURVE('',#6205,#6205,#1803,.T.);
#7839=EDGE_CURVE('',#6206,#6207,#371,.T.);
#7840=EDGE_CURVE('',#6207,#6206,#372,.T.);
#7841=EDGE_CURVE('',#6207,#6208,#4511,.T.);
#7842=EDGE_CURVE('',#6208,#6208,#1804,.T.);
#7843=EDGE_CURVE('',#6208,#6209,#4512,.T.);
#7844=EDGE_CURVE('',#6209,#6209,#1805,.T.);
#7845=EDGE_CURVE('',#6210,#6211,#4513,.T.);
#7846=EDGE_CURVE('',#6211,#6211,#1806,.T.);
#7847=EDGE_CURVE('',#6211,#6212,#4514,.T.);
#7848=EDGE_CURVE('',#6213,#6212,#373,.T.);
#7849=EDGE_CURVE('',#6214,#6213,#374,.T.);
#7850=EDGE_CURVE('',#6214,#6215,#4515,.T.);
#7851=EDGE_CURVE('',#6215,#6215,#1807,.T.);
#7852=EDGE_CURVE('',#6212,#6214,#375,.T.);
#7853=EDGE_CURVE('',#6215,#6216,#4516,.T.);
#7854=EDGE_CURVE('',#6217,#6216,#1808,.T.);
#7855=EDGE_CURVE('',#6218,#6217,#376,.T.);
#7856=EDGE_CURVE('',#6216,#6218,#1809,.T.);
#7857=EDGE_CURVE('',#6219,#6218,#4517,.T.);
#7858=EDGE_CURVE('',#6220,#6219,#4518,.T.);
#7859=EDGE_CURVE('',#6221,#6220,#4519,.T.);
#7860=EDGE_CURVE('',#6221,#6222,#1810,.T.);
#7861=EDGE_CURVE('',#6222,#6223,#1811,.T.);
#7862=EDGE_CURVE('',#6224,#6223,#4520,.T.);
#7863=EDGE_CURVE('',#6224,#6225,#1812,.T.);
#7864=EDGE_CURVE('',#6225,#6226,#1813,.T.);
#7865=EDGE_CURVE('',#6172,#6226,#4521,.T.);
#7866=EDGE_CURVE('',#6227,#6171,#4522,.T.);
#7867=EDGE_CURVE('',#6227,#6228,#1814,.T.);
#7868=EDGE_CURVE('',#6228,#6229,#1815,.T.);
#7869=EDGE_CURVE('',#6217,#6229,#4523,.T.);
#7870=EDGE_CURVE('',#6230,#6231,#4524,.T.);
#7871=EDGE_CURVE('',#6231,#6232,#4525,.T.);
#7872=EDGE_CURVE('',#6232,#6233,#4526,.T.);
#7873=EDGE_CURVE('',#6233,#6230,#4527,.T.);
#7874=EDGE_CURVE('',#6234,#6235,#4528,.T.);
#7875=EDGE_CURVE('',#6235,#6236,#4529,.T.);
#7876=EDGE_CURVE('',#6236,#6237,#4530,.T.);
#7877=EDGE_CURVE('',#6237,#6234,#4531,.T.);
#7878=EDGE_CURVE('',#6238,#6239,#4532,.T.);
#7879=EDGE_CURVE('',#6239,#6240,#4533,.T.);
#7880=EDGE_CURVE('',#6240,#6241,#4534,.T.);
#7881=EDGE_CURVE('',#6241,#6238,#4535,.T.);
#7882=EDGE_CURVE('',#6242,#6243,#4536,.T.);
#7883=EDGE_CURVE('',#6243,#6244,#4537,.T.);
#7884=EDGE_CURVE('',#6244,#6245,#4538,.T.);
#7885=EDGE_CURVE('',#6245,#6242,#4539,.T.);
#7886=EDGE_CURVE('',#6246,#6247,#4540,.T.);
#7887=EDGE_CURVE('',#6247,#6248,#4541,.T.);
#7888=EDGE_CURVE('',#6248,#6249,#4542,.T.);
#7889=EDGE_CURVE('',#6249,#6246,#4543,.T.);
#7890=EDGE_CURVE('',#6250,#6251,#4544,.T.);
#7891=EDGE_CURVE('',#6251,#6252,#4545,.T.);
#7892=EDGE_CURVE('',#6252,#6253,#4546,.T.);
#7893=EDGE_CURVE('',#6253,#6250,#4547,.T.);
#7894=EDGE_CURVE('',#6254,#6255,#4548,.T.);
#7895=EDGE_CURVE('',#6255,#6255,#1816,.T.);
#7896=EDGE_CURVE('',#6255,#6256,#4549,.T.);
#7897=EDGE_CURVE('',#6256,#6256,#1817,.T.);
#7898=EDGE_CURVE('',#6257,#6258,#377,.T.);
#7899=EDGE_CURVE('',#6258,#6257,#378,.T.);
#7900=EDGE_CURVE('',#6256,#6228,#4550,.T.);
#7901=EDGE_CURVE('',#6229,#6227,#379,.T.);
#7902=EDGE_CURVE('',#6136,#6134,#380,.T.);
#7903=EDGE_CURVE('',#6133,#6131,#381,.T.);
#7904=EDGE_CURVE('',#6130,#6219,#1818,.T.);
#7905=EDGE_CURVE('',#6259,#6260,#4551,.T.);
#7906=EDGE_CURVE('',#6260,#6260,#1819,.T.);
#7907=EDGE_CURVE('',#6260,#6261,#4552,.T.);
#7908=EDGE_CURVE('',#6261,#6261,#1820,.T.);
#7909=EDGE_CURVE('',#6261,#6222,#4553,.T.);
#7910=EDGE_CURVE('',#6223,#6221,#382,.T.);
#7911=EDGE_CURVE('',#6220,#6067,#1821,.T.);
#7912=EDGE_CURVE('',#6226,#6224,#383,.T.);
#7913=EDGE_CURVE('',#6262,#6263,#4554,.T.);
#7914=EDGE_CURVE('',#6263,#6263,#1822,.T.);
#7915=EDGE_CURVE('',#6263,#6264,#4555,.T.);
#7916=EDGE_CURVE('',#6264,#6264,#1823,.T.);
#7917=EDGE_CURVE('',#6264,#6225,#4556,.T.);
#7918=EDGE_CURVE('',#6265,#6266,#4557,.T.);
#7919=EDGE_CURVE('',#6266,#6266,#1824,.T.);
#7920=EDGE_CURVE('',#6266,#6267,#4558,.T.);
#7921=EDGE_CURVE('',#6267,#6267,#1825,.T.);
#7922=EDGE_CURVE('',#6267,#6205,#4559,.T.);
#7923=EDGE_CURVE('',#6268,#6269,#4560,.T.);
#7924=EDGE_CURVE('',#6269,#6269,#1826,.T.);
#7925=EDGE_CURVE('',#6269,#6270,#4561,.T.);
#7926=EDGE_CURVE('',#6270,#6270,#1827,.T.);
#7927=EDGE_CURVE('',#6270,#6271,#4562,.T.);
#7928=EDGE_CURVE('',#6271,#6271,#1828,.T.);
#7929=EDGE_CURVE('',#6272,#6273,#4563,.T.);
#7930=EDGE_CURVE('',#6273,#6273,#1829,.T.);
#7931=EDGE_CURVE('',#6273,#6274,#4564,.T.);
#7932=EDGE_CURVE('',#6274,#6274,#1830,.T.);
#7933=EDGE_CURVE('',#6274,#6204,#4565,.T.);
#7934=EDGE_CURVE('',#6275,#6276,#4566,.T.);
#7935=EDGE_CURVE('',#6276,#6276,#1831,.T.);
#7936=EDGE_CURVE('',#6276,#6277,#4567,.T.);
#7937=EDGE_CURVE('',#6277,#6277,#1832,.T.);
#7938=EDGE_CURVE('',#6277,#6278,#4568,.T.);
#7939=EDGE_CURVE('',#6278,#6278,#1833,.T.);
#7940=EDGE_CURVE('',#6279,#6280,#4569,.T.);
#7941=EDGE_CURVE('',#6280,#6280,#1834,.T.);
#7942=EDGE_CURVE('',#6280,#6281,#4570,.T.);
#7943=EDGE_CURVE('',#6281,#6281,#1835,.T.);
#7944=EDGE_CURVE('',#6281,#6203,#4571,.T.);
#7945=EDGE_CURVE('',#6282,#6283,#4572,.T.);
#7946=EDGE_CURVE('',#6283,#6283,#1836,.T.);
#7947=EDGE_CURVE('',#6283,#6284,#4573,.T.);
#7948=EDGE_CURVE('',#6284,#6284,#1837,.T.);
#7949=EDGE_CURVE('',#6284,#6285,#4574,.T.);
#7950=EDGE_CURVE('',#6285,#6285,#1838,.T.);
#7951=EDGE_CURVE('',#6286,#6287,#4575,.T.);
#7952=EDGE_CURVE('',#6287,#6287,#1839,.T.);
#7953=EDGE_CURVE('',#6287,#6288,#4576,.T.);
#7954=EDGE_CURVE('',#6288,#6288,#1840,.T.);
#7955=EDGE_CURVE('',#6288,#6202,#4577,.T.);
#7956=EDGE_CURVE('',#6289,#6290,#4578,.T.);
#7957=EDGE_CURVE('',#6290,#6290,#1841,.T.);
#7958=EDGE_CURVE('',#6290,#6291,#4579,.T.);
#7959=EDGE_CURVE('',#6291,#6291,#1842,.T.);
#7960=EDGE_CURVE('',#6291,#6292,#4580,.T.);
#7961=EDGE_CURVE('',#6292,#6292,#1843,.T.);
#7962=EDGE_CURVE('',#6293,#6294,#4581,.T.);
#7963=EDGE_CURVE('',#6294,#6294,#1844,.T.);
#7964=EDGE_CURVE('',#6294,#6295,#4582,.T.);
#7965=EDGE_CURVE('',#6295,#6295,#1845,.T.);
#7966=EDGE_CURVE('',#6295,#6145,#4583,.T.);
#7967=EDGE_CURVE('',#6296,#6297,#4584,.T.);
#7968=EDGE_CURVE('',#6297,#6297,#1846,.T.);
#7969=EDGE_CURVE('',#6297,#6298,#4585,.T.);
#7970=EDGE_CURVE('',#6298,#6298,#1847,.T.);
#7971=EDGE_CURVE('',#6298,#6144,#4586,.T.);
#7972=EDGE_CURVE('',#6299,#6300,#4587,.T.);
#7973=EDGE_CURVE('',#6300,#6300,#1848,.T.);
#7974=EDGE_CURVE('',#6300,#6301,#4588,.T.);
#7975=EDGE_CURVE('',#6301,#6301,#1849,.T.);
#7976=EDGE_CURVE('',#6301,#6132,#4589,.T.);
#7977=EDGE_CURVE('',#6302,#6303,#4590,.T.);
#7978=EDGE_CURVE('',#6303,#6303,#1850,.T.);
#7979=EDGE_CURVE('',#6303,#6257,#4591,.T.);
#7980=EDGE_CURVE('',#6258,#6304,#4592,.T.);
#7981=EDGE_CURVE('',#6304,#6304,#1851,.T.);
#7982=EDGE_CURVE('',#6304,#6135,#4593,.T.);
#7983=EDGE_CURVE('',#6305,#6305,#1852,.T.);
#7984=EDGE_CURVE('',#6305,#6306,#4594,.T.);
#7985=EDGE_CURVE('',#6306,#6306,#1853,.T.);
#7986=EDGE_CURVE('',#6306,#6307,#4595,.T.);
#7987=EDGE_CURVE('',#6307,#6307,#1854,.T.);
#7988=EDGE_CURVE('',#6308,#6308,#1855,.T.);
#7989=EDGE_CURVE('',#6308,#6309,#4596,.T.);
#7990=EDGE_CURVE('',#6309,#6309,#1856,.T.);
#7991=EDGE_CURVE('',#6309,#6310,#4597,.T.);
#7992=EDGE_CURVE('',#6310,#6310,#1857,.T.);
#7993=EDGE_CURVE('',#6311,#6311,#1858,.T.);
#7994=EDGE_CURVE('',#6311,#6312,#4598,.T.);
#7995=EDGE_CURVE('',#6312,#6312,#1859,.T.);
#7996=EDGE_CURVE('',#6312,#6313,#4599,.T.);
#7997=EDGE_CURVE('',#6313,#6313,#1860,.T.);
#7998=EDGE_CURVE('',#6314,#6314,#1861,.T.);
#7999=EDGE_CURVE('',#6314,#6315,#4600,.T.);
#8000=EDGE_CURVE('',#6315,#6315,#1862,.T.);
#8001=EDGE_CURVE('',#6315,#6316,#4601,.T.);
#8002=EDGE_CURVE('',#6316,#6316,#1863,.T.);
#8003=EDGE_CURVE('',#6317,#6059,#4602,.T.);
#8004=EDGE_CURVE('',#6056,#6317,#4603,.T.);
#8005=EDGE_CURVE('',#6060,#6317,#4604,.T.);
#8006=EDGE_CURVE('',#6125,#6318,#4605,.T.);
#8007=EDGE_CURVE('',#6129,#6318,#4606,.T.);
#8008=EDGE_CURVE('',#6318,#6319,#4607,.T.);
#8009=EDGE_CURVE('',#6124,#6319,#4608,.T.);
#8010=EDGE_CURVE('',#6319,#6142,#4609,.T.);
#8011=EDGE_CURVE('',#6320,#6141,#1864,.T.);
#8012=EDGE_CURVE('',#6320,#6321,#4610,.T.);
#8013=EDGE_CURVE('',#6321,#6322,#4611,.T.);
#8014=EDGE_CURVE('',#6322,#6323,#4612,.T.);
#8015=EDGE_CURVE('',#6323,#6324,#4613,.T.);
#8016=EDGE_CURVE('',#6324,#6325,#4614,.T.);
#8017=EDGE_CURVE('',#6061,#6325,#1865,.T.);
#8018=EDGE_CURVE('',#6326,#6326,#1866,.T.);
#8019=EDGE_CURVE('',#6327,#6063,#4615,.T.);
#8020=EDGE_CURVE('',#6328,#6327,#4616,.T.);
#8021=EDGE_CURVE('',#6328,#6064,#4617,.T.);
#8022=EDGE_CURVE('',#6329,#6328,#4618,.T.);
#8023=EDGE_CURVE('',#6054,#6329,#4619,.T.);
#8024=EDGE_CURVE('',#6329,#6173,#4620,.T.);
#8025=EDGE_CURVE('',#6330,#6327,#4621,.T.);
#8026=EDGE_CURVE('',#6190,#6330,#4622,.T.);
#8027=EDGE_CURVE('',#6331,#6184,#4623,.T.);
#8028=EDGE_CURVE('',#6332,#6331,#4624,.T.);
#8029=EDGE_CURVE('',#6333,#6332,#4625,.T.);
#8030=EDGE_CURVE('',#6333,#6128,#4626,.T.);
#8031=EDGE_CURVE('',#6182,#6170,#4627,.T.);
#8032=EDGE_CURVE('',#6139,#6332,#4628,.T.);
#8033=EDGE_CURVE('',#6138,#6333,#4629,.T.);
#8034=EDGE_CURVE('',#6334,#6330,#1867,.T.);
#8035=EDGE_CURVE('',#6334,#6188,#4630,.T.);
#8036=EDGE_CURVE('',#6335,#6186,#4631,.T.);
#8037=EDGE_CURVE('',#6331,#6335,#1868,.T.);
#8038=EDGE_CURVE('',#6336,#6062,#1869,.T.);
#8039=EDGE_CURVE('',#6336,#6337,#4632,.T.);
#8040=EDGE_CURVE('',#6337,#6338,#4633,.T.);
#8041=EDGE_CURVE('',#6338,#6339,#4634,.T.);
#8042=EDGE_CURVE('',#6339,#6340,#4635,.T.);
#8043=EDGE_CURVE('',#6340,#6341,#4636,.T.);
#8044=EDGE_CURVE('',#6140,#6341,#1870,.T.);
#8045=EDGE_CURVE('',#6335,#6334,#1871,.T.);
#8046=EDGE_CURVE('',#6339,#6322,#4637,.T.);
#8047=EDGE_CURVE('',#6340,#6321,#4638,.T.);
#8048=EDGE_CURVE('',#6324,#6337,#4639,.T.);
#8049=EDGE_CURVE('',#6323,#6338,#4640,.T.);
#8050=EDGE_CURVE('',#6325,#6336,#4641,.T.);
#8051=EDGE_CURVE('',#6341,#6320,#4642,.T.);
#8052=EDGE_CURVE('',#6250,#6342,#4643,.T.);
#8053=EDGE_CURVE('',#6342,#6343,#4644,.T.);
#8054=EDGE_CURVE('',#6251,#6343,#4645,.T.);
#8055=EDGE_CURVE('',#6253,#6344,#4646,.T.);
#8056=EDGE_CURVE('',#6344,#6342,#4647,.T.);
#8057=EDGE_CURVE('',#6252,#6345,#4648,.T.);
#8058=EDGE_CURVE('',#6345,#6344,#4649,.T.);
#8059=EDGE_CURVE('',#6343,#6345,#4650,.T.);
#8060=EDGE_CURVE('',#6246,#6346,#4651,.T.);
#8061=EDGE_CURVE('',#6346,#6347,#4652,.T.);
#8062=EDGE_CURVE('',#6247,#6347,#4653,.T.);
#8063=EDGE_CURVE('',#6249,#6348,#4654,.T.);
#8064=EDGE_CURVE('',#6348,#6346,#4655,.T.);
#8065=EDGE_CURVE('',#6248,#6349,#4656,.T.);
#8066=EDGE_CURVE('',#6349,#6348,#4657,.T.);
#8067=EDGE_CURVE('',#6347,#6349,#4658,.T.);
#8068=EDGE_CURVE('',#6242,#6350,#4659,.T.);
#8069=EDGE_CURVE('',#6350,#6351,#4660,.T.);
#8070=EDGE_CURVE('',#6243,#6351,#4661,.T.);
#8071=EDGE_CURVE('',#6245,#6352,#4662,.T.);
#8072=EDGE_CURVE('',#6352,#6350,#4663,.T.);
#8073=EDGE_CURVE('',#6244,#6353,#4664,.T.);
#8074=EDGE_CURVE('',#6353,#6352,#4665,.T.);
#8075=EDGE_CURVE('',#6351,#6353,#4666,.T.);
#8076=EDGE_CURVE('',#6238,#6354,#4667,.T.);
#8077=EDGE_CURVE('',#6354,#6355,#4668,.T.);
#8078=EDGE_CURVE('',#6239,#6355,#4669,.T.);
#8079=EDGE_CURVE('',#6241,#6356,#4670,.T.);
#8080=EDGE_CURVE('',#6356,#6354,#4671,.T.);
#8081=EDGE_CURVE('',#6240,#6357,#4672,.T.);
#8082=EDGE_CURVE('',#6357,#6356,#4673,.T.);
#8083=EDGE_CURVE('',#6355,#6357,#4674,.T.);
#8084=EDGE_CURVE('',#6234,#6358,#4675,.T.);
#8085=EDGE_CURVE('',#6358,#6359,#4676,.T.);
#8086=EDGE_CURVE('',#6235,#6359,#4677,.T.);
#8087=EDGE_CURVE('',#6237,#6360,#4678,.T.);
#8088=EDGE_CURVE('',#6360,#6358,#4679,.T.);
#8089=EDGE_CURVE('',#6236,#6361,#4680,.T.);
#8090=EDGE_CURVE('',#6361,#6360,#4681,.T.);
#8091=EDGE_CURVE('',#6359,#6361,#4682,.T.);
#8092=EDGE_CURVE('',#6230,#6362,#4683,.T.);
#8093=EDGE_CURVE('',#6362,#6363,#4684,.T.);
#8094=EDGE_CURVE('',#6231,#6363,#4685,.T.);
#8095=EDGE_CURVE('',#6233,#6364,#4686,.T.);
#8096=EDGE_CURVE('',#6364,#6362,#4687,.T.);
#8097=EDGE_CURVE('',#6232,#6365,#4688,.T.);
#8098=EDGE_CURVE('',#6365,#6364,#4689,.T.);
#8099=EDGE_CURVE('',#6363,#6365,#4690,.T.);
#8100=EDGE_CURVE('',#6068,#6366,#4691,.T.);
#8101=EDGE_CURVE('',#6366,#6366,#1872,.T.);
#8102=EDGE_CURVE('',#6367,#6367,#1873,.T.);
#8103=EDGE_CURVE('',#6367,#6368,#4692,.T.);
#8104=EDGE_CURVE('',#6368,#6368,#1874,.T.);
#8105=EDGE_CURVE('',#6369,#6369,#1875,.T.);
#8106=EDGE_CURVE('',#6369,#6370,#4693,.T.);
#8107=EDGE_CURVE('',#6370,#6370,#1876,.T.);
#8108=EDGE_CURVE('',#6371,#6371,#1877,.T.);
#8109=EDGE_CURVE('',#6371,#6372,#4694,.T.);
#8110=EDGE_CURVE('',#6373,#6372,#384,.T.);
#8111=EDGE_CURVE('',#6374,#6373,#385,.T.);
#8112=EDGE_CURVE('',#6374,#6375,#4695,.T.);
#8113=EDGE_CURVE('',#6375,#6375,#1878,.T.);
#8114=EDGE_CURVE('',#6372,#6374,#386,.T.);
#8115=EDGE_CURVE('',#6376,#6376,#1879,.T.);
#8116=EDGE_CURVE('',#6376,#6377,#4696,.T.);
#8117=EDGE_CURVE('',#6377,#6377,#1880,.T.);
#8118=EDGE_CURVE('',#6378,#6378,#1881,.T.);
#8119=EDGE_CURVE('',#6378,#6379,#4697,.T.);
#8120=EDGE_CURVE('',#6379,#6379,#1882,.T.);
#8121=EDGE_CURVE('',#6380,#6380,#1883,.T.);
#8122=EDGE_CURVE('',#6380,#6143,#4698,.T.);
#8123=EDGE_CURVE('',#6326,#6381,#4699,.T.);
#8124=EDGE_CURVE('',#6381,#6381,#1884,.T.);
#8125=EDGE_CURVE('',#6382,#6382,#1885,.T.);
#8126=EDGE_CURVE('',#6382,#6383,#4700,.T.);
#8127=EDGE_CURVE('',#6383,#6383,#1886,.T.);
#8128=EDGE_CURVE('',#6384,#6384,#1887,.T.);
#8129=EDGE_CURVE('',#6384,#6385,#4701,.T.);
#8130=EDGE_CURVE('',#6385,#6385,#1888,.T.);
#8131=EDGE_CURVE('',#6385,#6201,#4702,.T.);
#9851=ORIENTED_EDGE('',*,*,#7547,.F.);
#9852=ORIENTED_EDGE('',*,*,#7548,.T.);
#9853=ORIENTED_EDGE('',*,*,#7549,.T.);
#9854=ORIENTED_EDGE('',*,*,#7550,.F.);
#9855=ORIENTED_EDGE('',*,*,#7551,.F.);
#9856=ORIENTED_EDGE('',*,*,#7552,.T.);
#9857=ORIENTED_EDGE('',*,*,#7553,.T.);
#9858=ORIENTED_EDGE('',*,*,#7548,.F.);
#9859=ORIENTED_EDGE('',*,*,#7554,.F.);
#9860=ORIENTED_EDGE('',*,*,#7555,.T.);
#9861=ORIENTED_EDGE('',*,*,#7556,.T.);
#9862=ORIENTED_EDGE('',*,*,#7552,.F.);
#9863=ORIENTED_EDGE('',*,*,#7557,.F.);
#9864=ORIENTED_EDGE('',*,*,#7550,.T.);
#9865=ORIENTED_EDGE('',*,*,#7558,.T.);
#9866=ORIENTED_EDGE('',*,*,#7555,.F.);
#9867=ORIENTED_EDGE('',*,*,#7558,.F.);
#9868=ORIENTED_EDGE('',*,*,#7549,.F.);
#9869=ORIENTED_EDGE('',*,*,#7553,.F.);
#9870=ORIENTED_EDGE('',*,*,#7556,.F.);
#9871=ORIENTED_EDGE('',*,*,#7559,.F.);
#9872=ORIENTED_EDGE('',*,*,#7560,.F.);
#9873=ORIENTED_EDGE('',*,*,#7561,.T.);
#9874=ORIENTED_EDGE('',*,*,#7562,.T.);
#9875=ORIENTED_EDGE('',*,*,#7563,.F.);
#9876=ORIENTED_EDGE('',*,*,#7562,.F.);
#9877=ORIENTED_EDGE('',*,*,#7564,.F.);
#9878=ORIENTED_EDGE('',*,*,#7565,.F.);
#9879=ORIENTED_EDGE('',*,*,#7566,.F.);
#9880=ORIENTED_EDGE('',*,*,#7567,.F.);
#9881=ORIENTED_EDGE('',*,*,#7568,.F.);
#9882=ORIENTED_EDGE('',*,*,#7569,.T.);
#9883=ORIENTED_EDGE('',*,*,#7564,.T.);
#9884=ORIENTED_EDGE('',*,*,#7561,.F.);
#9885=ORIENTED_EDGE('',*,*,#7570,.F.);
#9886=ORIENTED_EDGE('',*,*,#7571,.T.);
#9887=ORIENTED_EDGE('',*,*,#7565,.T.);
#9888=ORIENTED_EDGE('',*,*,#7569,.F.);
#9889=ORIENTED_EDGE('',*,*,#7572,.F.);
#9890=ORIENTED_EDGE('',*,*,#7566,.T.);
#9891=ORIENTED_EDGE('',*,*,#7571,.F.);
#9892=ORIENTED_EDGE('',*,*,#7573,.F.);
#9893=ORIENTED_EDGE('',*,*,#7574,.F.);
#9894=ORIENTED_EDGE('',*,*,#7575,.T.);
#9895=ORIENTED_EDGE('',*,*,#7576,.T.);
#9896=ORIENTED_EDGE('',*,*,#7577,.F.);
#9897=ORIENTED_EDGE('',*,*,#7578,.F.);
#9898=ORIENTED_EDGE('',*,*,#7579,.T.);
#9899=ORIENTED_EDGE('',*,*,#7580,.T.);
#9900=ORIENTED_EDGE('',*,*,#7575,.F.);
#9901=ORIENTED_EDGE('',*,*,#7581,.F.);
#9902=ORIENTED_EDGE('',*,*,#7582,.T.);
#9903=ORIENTED_EDGE('',*,*,#7583,.T.);
#9904=ORIENTED_EDGE('',*,*,#7579,.F.);
#9905=ORIENTED_EDGE('',*,*,#7584,.F.);
#9906=ORIENTED_EDGE('',*,*,#7577,.T.);
#9907=ORIENTED_EDGE('',*,*,#7585,.T.);
#9908=ORIENTED_EDGE('',*,*,#7582,.F.);
#9909=ORIENTED_EDGE('',*,*,#7585,.F.);
#9910=ORIENTED_EDGE('',*,*,#7576,.F.);
#9911=ORIENTED_EDGE('',*,*,#7580,.F.);
#9912=ORIENTED_EDGE('',*,*,#7583,.F.);
#9913=ORIENTED_EDGE('',*,*,#7586,.F.);
#9914=ORIENTED_EDGE('',*,*,#7587,.T.);
#9915=ORIENTED_EDGE('',*,*,#7588,.T.);
#9916=ORIENTED_EDGE('',*,*,#7589,.F.);
#9917=ORIENTED_EDGE('',*,*,#7590,.F.);
#9918=ORIENTED_EDGE('',*,*,#7591,.T.);
#9919=ORIENTED_EDGE('',*,*,#7592,.T.);
#9920=ORIENTED_EDGE('',*,*,#7587,.F.);
#9921=ORIENTED_EDGE('',*,*,#7593,.F.);
#9922=ORIENTED_EDGE('',*,*,#7594,.T.);
#9923=ORIENTED_EDGE('',*,*,#7595,.T.);
#9924=ORIENTED_EDGE('',*,*,#7591,.F.);
#9925=ORIENTED_EDGE('',*,*,#7596,.F.);
#9926=ORIENTED_EDGE('',*,*,#7589,.T.);
#9927=ORIENTED_EDGE('',*,*,#7597,.T.);
#9928=ORIENTED_EDGE('',*,*,#7594,.F.);
#9929=ORIENTED_EDGE('',*,*,#7597,.F.);
#9930=ORIENTED_EDGE('',*,*,#7588,.F.);
#9931=ORIENTED_EDGE('',*,*,#7592,.F.);
#9932=ORIENTED_EDGE('',*,*,#7595,.F.);
#9933=ORIENTED_EDGE('',*,*,#7598,.F.);
#9934=ORIENTED_EDGE('',*,*,#7599,.T.);
#9935=ORIENTED_EDGE('',*,*,#7600,.T.);
#9936=ORIENTED_EDGE('',*,*,#7601,.F.);
#9937=ORIENTED_EDGE('',*,*,#7602,.F.);
#9938=ORIENTED_EDGE('',*,*,#7603,.T.);
#9939=ORIENTED_EDGE('',*,*,#7604,.T.);
#9940=ORIENTED_EDGE('',*,*,#7599,.F.);
#9941=ORIENTED_EDGE('',*,*,#7605,.F.);
#9942=ORIENTED_EDGE('',*,*,#7606,.T.);
#9943=ORIENTED_EDGE('',*,*,#7607,.T.);
#9944=ORIENTED_EDGE('',*,*,#7603,.F.);
#9945=ORIENTED_EDGE('',*,*,#7608,.F.);
#9946=ORIENTED_EDGE('',*,*,#7601,.T.);
#9947=ORIENTED_EDGE('',*,*,#7609,.T.);
#9948=ORIENTED_EDGE('',*,*,#7606,.F.);
#9949=ORIENTED_EDGE('',*,*,#7609,.F.);
#9950=ORIENTED_EDGE('',*,*,#7600,.F.);
#9951=ORIENTED_EDGE('',*,*,#7604,.F.);
#9952=ORIENTED_EDGE('',*,*,#7607,.F.);
#9953=ORIENTED_EDGE('',*,*,#7610,.F.);
#9954=ORIENTED_EDGE('',*,*,#7611,.T.);
#9955=ORIENTED_EDGE('',*,*,#7612,.F.);
#9956=ORIENTED_EDGE('',*,*,#7613,.F.);
#9957=ORIENTED_EDGE('',*,*,#7614,.F.);
#9958=ORIENTED_EDGE('',*,*,#7615,.F.);
#9959=ORIENTED_EDGE('',*,*,#7616,.T.);
#9960=ORIENTED_EDGE('',*,*,#7617,.T.);
#9961=ORIENTED_EDGE('',*,*,#7618,.F.);
#9962=ORIENTED_EDGE('',*,*,#7619,.T.);
#9963=ORIENTED_EDGE('',*,*,#7620,.T.);
#9964=ORIENTED_EDGE('',*,*,#7616,.F.);
#9965=ORIENTED_EDGE('',*,*,#7621,.F.);
#9966=ORIENTED_EDGE('',*,*,#7612,.T.);
#9967=ORIENTED_EDGE('',*,*,#7622,.T.);
#9968=ORIENTED_EDGE('',*,*,#7619,.F.);
#9969=ORIENTED_EDGE('',*,*,#7623,.F.);
#9970=ORIENTED_EDGE('',*,*,#7624,.F.);
#9971=ORIENTED_EDGE('',*,*,#7617,.F.);
#9972=ORIENTED_EDGE('',*,*,#7620,.F.);
#9973=ORIENTED_EDGE('',*,*,#7622,.F.);
#9974=ORIENTED_EDGE('',*,*,#7611,.F.);
#9975=ORIENTED_EDGE('',*,*,#7559,.T.);
#9976=ORIENTED_EDGE('',*,*,#7563,.T.);
#9977=ORIENTED_EDGE('',*,*,#7625,.T.);
#9978=ORIENTED_EDGE('',*,*,#7626,.T.);
#9979=ORIENTED_EDGE('',*,*,#7627,.T.);
#9980=ORIENTED_EDGE('',*,*,#7628,.F.);
#9981=ORIENTED_EDGE('',*,*,#7567,.T.);
#9982=ORIENTED_EDGE('',*,*,#7572,.T.);
#9983=ORIENTED_EDGE('',*,*,#7629,.F.);
#9984=ORIENTED_EDGE('',*,*,#7630,.F.);
#9985=ORIENTED_EDGE('',*,*,#7631,.F.);
#9986=ORIENTED_EDGE('',*,*,#7625,.F.);
#9987=ORIENTED_EDGE('',*,*,#7560,.T.);
#9988=ORIENTED_EDGE('',*,*,#7628,.T.);
#9989=ORIENTED_EDGE('',*,*,#7632,.T.);
#9990=ORIENTED_EDGE('',*,*,#7633,.F.);
#9991=ORIENTED_EDGE('',*,*,#7634,.F.);
#9992=ORIENTED_EDGE('',*,*,#7635,.F.);
#9993=ORIENTED_EDGE('',*,*,#7636,.T.);
#9994=ORIENTED_EDGE('',*,*,#7637,.T.);
#9995=ORIENTED_EDGE('',*,*,#7613,.T.);
#9996=ORIENTED_EDGE('',*,*,#7621,.T.);
#9997=ORIENTED_EDGE('',*,*,#7618,.T.);
#9998=ORIENTED_EDGE('',*,*,#7615,.T.);
#9999=ORIENTED_EDGE('',*,*,#7638,.T.);
#10000=ORIENTED_EDGE('',*,*,#7639,.F.);
#10001=ORIENTED_EDGE('',*,*,#7640,.F.);
#10002=ORIENTED_EDGE('',*,*,#7641,.F.);
#10003=ORIENTED_EDGE('',*,*,#7629,.T.);
#10004=ORIENTED_EDGE('',*,*,#7573,.T.);
#10005=ORIENTED_EDGE('',*,*,#7570,.T.);
#10006=ORIENTED_EDGE('',*,*,#7568,.T.);
#10007=ORIENTED_EDGE('',*,*,#7642,.T.);
#10008=ORIENTED_EDGE('',*,*,#7598,.T.);
#10009=ORIENTED_EDGE('',*,*,#7608,.T.);
#10010=ORIENTED_EDGE('',*,*,#7605,.T.);
#10011=ORIENTED_EDGE('',*,*,#7602,.T.);
#10012=ORIENTED_EDGE('',*,*,#7586,.T.);
#10013=ORIENTED_EDGE('',*,*,#7596,.T.);
#10014=ORIENTED_EDGE('',*,*,#7593,.T.);
#10015=ORIENTED_EDGE('',*,*,#7590,.T.);
#10016=ORIENTED_EDGE('',*,*,#7574,.T.);
#10017=ORIENTED_EDGE('',*,*,#7584,.T.);
#10018=ORIENTED_EDGE('',*,*,#7581,.T.);
#10019=ORIENTED_EDGE('',*,*,#7578,.T.);
#10020=ORIENTED_EDGE('',*,*,#7547,.T.);
#10021=ORIENTED_EDGE('',*,*,#7557,.T.);
#10022=ORIENTED_EDGE('',*,*,#7554,.T.);
#10023=ORIENTED_EDGE('',*,*,#7551,.T.);
#10024=ORIENTED_EDGE('',*,*,#7643,.F.);
#10025=ORIENTED_EDGE('',*,*,#7644,.T.);
#10026=ORIENTED_EDGE('',*,*,#7645,.T.);
#10027=ORIENTED_EDGE('',*,*,#7646,.F.);
#10028=ORIENTED_EDGE('',*,*,#7647,.F.);
#10029=ORIENTED_EDGE('',*,*,#7648,.T.);
#10030=ORIENTED_EDGE('',*,*,#7649,.T.);
#10031=ORIENTED_EDGE('',*,*,#7644,.F.);
#10032=ORIENTED_EDGE('',*,*,#7650,.F.);
#10033=ORIENTED_EDGE('',*,*,#7651,.T.);
#10034=ORIENTED_EDGE('',*,*,#7652,.T.);
#10035=ORIENTED_EDGE('',*,*,#7648,.F.);
#10036=ORIENTED_EDGE('',*,*,#7653,.F.);
#10037=ORIENTED_EDGE('',*,*,#7646,.T.);
#10038=ORIENTED_EDGE('',*,*,#7654,.T.);
#10039=ORIENTED_EDGE('',*,*,#7651,.F.);
#10040=ORIENTED_EDGE('',*,*,#7654,.F.);
#10041=ORIENTED_EDGE('',*,*,#7645,.F.);
#10042=ORIENTED_EDGE('',*,*,#7649,.F.);
#10043=ORIENTED_EDGE('',*,*,#7652,.F.);
#10044=ORIENTED_EDGE('',*,*,#7655,.F.);
#10045=ORIENTED_EDGE('',*,*,#7656,.T.);
#10046=ORIENTED_EDGE('',*,*,#7657,.F.);
#10047=ORIENTED_EDGE('',*,*,#7658,.F.);
#10048=ORIENTED_EDGE('',*,*,#7659,.F.);
#10049=ORIENTED_EDGE('',*,*,#7660,.T.);
#10050=ORIENTED_EDGE('',*,*,#7661,.T.);
#10051=ORIENTED_EDGE('',*,*,#7662,.F.);
#10052=ORIENTED_EDGE('',*,*,#7663,.F.);
#10053=ORIENTED_EDGE('',*,*,#7657,.T.);
#10054=ORIENTED_EDGE('',*,*,#7664,.T.);
#10055=ORIENTED_EDGE('',*,*,#7660,.F.);
#10056=ORIENTED_EDGE('',*,*,#7665,.F.);
#10057=ORIENTED_EDGE('',*,*,#7666,.F.);
#10058=ORIENTED_EDGE('',*,*,#7662,.T.);
#10059=ORIENTED_EDGE('',*,*,#7667,.T.);
#10060=ORIENTED_EDGE('',*,*,#7668,.F.);
#10061=ORIENTED_EDGE('',*,*,#7669,.F.);
#10062=ORIENTED_EDGE('',*,*,#7667,.F.);
#10063=ORIENTED_EDGE('',*,*,#7661,.F.);
#10064=ORIENTED_EDGE('',*,*,#7664,.F.);
#10065=ORIENTED_EDGE('',*,*,#7656,.F.);
#10066=ORIENTED_EDGE('',*,*,#7670,.F.);
#10067=ORIENTED_EDGE('',*,*,#7671,.T.);
#10068=ORIENTED_EDGE('',*,*,#7672,.T.);
#10069=ORIENTED_EDGE('',*,*,#7673,.F.);
#10070=ORIENTED_EDGE('',*,*,#7674,.F.);
#10071=ORIENTED_EDGE('',*,*,#7675,.T.);
#10072=ORIENTED_EDGE('',*,*,#7676,.T.);
#10073=ORIENTED_EDGE('',*,*,#7671,.F.);
#10074=ORIENTED_EDGE('',*,*,#7677,.F.);
#10075=ORIENTED_EDGE('',*,*,#7678,.T.);
#10076=ORIENTED_EDGE('',*,*,#7679,.T.);
#10077=ORIENTED_EDGE('',*,*,#7675,.F.);
#10078=ORIENTED_EDGE('',*,*,#7680,.F.);
#10079=ORIENTED_EDGE('',*,*,#7673,.T.);
#10080=ORIENTED_EDGE('',*,*,#7681,.T.);
#10081=ORIENTED_EDGE('',*,*,#7678,.F.);
#10082=ORIENTED_EDGE('',*,*,#7681,.F.);
#10083=ORIENTED_EDGE('',*,*,#7672,.F.);
#10084=ORIENTED_EDGE('',*,*,#7676,.F.);
#10085=ORIENTED_EDGE('',*,*,#7679,.F.);
#10086=ORIENTED_EDGE('',*,*,#7682,.F.);
#10087=ORIENTED_EDGE('',*,*,#7683,.T.);
#10088=ORIENTED_EDGE('',*,*,#7684,.T.);
#10089=ORIENTED_EDGE('',*,*,#7685,.F.);
#10090=ORIENTED_EDGE('',*,*,#7686,.F.);
#10091=ORIENTED_EDGE('',*,*,#7687,.T.);
#10092=ORIENTED_EDGE('',*,*,#7688,.T.);
#10093=ORIENTED_EDGE('',*,*,#7683,.F.);
#10094=ORIENTED_EDGE('',*,*,#7689,.F.);
#10095=ORIENTED_EDGE('',*,*,#7690,.T.);
#10096=ORIENTED_EDGE('',*,*,#7691,.T.);
#10097=ORIENTED_EDGE('',*,*,#7687,.F.);
#10098=ORIENTED_EDGE('',*,*,#7692,.F.);
#10099=ORIENTED_EDGE('',*,*,#7685,.T.);
#10100=ORIENTED_EDGE('',*,*,#7693,.T.);
#10101=ORIENTED_EDGE('',*,*,#7690,.F.);
#10102=ORIENTED_EDGE('',*,*,#7693,.F.);
#10103=ORIENTED_EDGE('',*,*,#7684,.F.);
#10104=ORIENTED_EDGE('',*,*,#7688,.F.);
#10105=ORIENTED_EDGE('',*,*,#7691,.F.);
#10106=ORIENTED_EDGE('',*,*,#7694,.F.);
#10107=ORIENTED_EDGE('',*,*,#7695,.T.);
#10108=ORIENTED_EDGE('',*,*,#7696,.T.);
#10109=ORIENTED_EDGE('',*,*,#7697,.F.);
#10110=ORIENTED_EDGE('',*,*,#7698,.F.);
#10111=ORIENTED_EDGE('',*,*,#7699,.T.);
#10112=ORIENTED_EDGE('',*,*,#7700,.T.);
#10113=ORIENTED_EDGE('',*,*,#7695,.F.);
#10114=ORIENTED_EDGE('',*,*,#7701,.F.);
#10115=ORIENTED_EDGE('',*,*,#7702,.T.);
#10116=ORIENTED_EDGE('',*,*,#7703,.T.);
#10117=ORIENTED_EDGE('',*,*,#7699,.F.);
#10118=ORIENTED_EDGE('',*,*,#7704,.F.);
#10119=ORIENTED_EDGE('',*,*,#7697,.T.);
#10120=ORIENTED_EDGE('',*,*,#7705,.T.);
#10121=ORIENTED_EDGE('',*,*,#7702,.F.);
#10122=ORIENTED_EDGE('',*,*,#7705,.F.);
#10123=ORIENTED_EDGE('',*,*,#7696,.F.);
#10124=ORIENTED_EDGE('',*,*,#7700,.F.);
#10125=ORIENTED_EDGE('',*,*,#7703,.F.);
#10126=ORIENTED_EDGE('',*,*,#7706,.F.);
#10127=ORIENTED_EDGE('',*,*,#7707,.T.);
#10128=ORIENTED_EDGE('',*,*,#7708,.F.);
#10129=ORIENTED_EDGE('',*,*,#7709,.F.);
#10130=ORIENTED_EDGE('',*,*,#7710,.F.);
#10131=ORIENTED_EDGE('',*,*,#7708,.T.);
#10132=ORIENTED_EDGE('',*,*,#7711,.T.);
#10133=ORIENTED_EDGE('',*,*,#7712,.F.);
#10134=ORIENTED_EDGE('',*,*,#7713,.F.);
#10135=ORIENTED_EDGE('',*,*,#7714,.F.);
#10136=ORIENTED_EDGE('',*,*,#7715,.T.);
#10137=ORIENTED_EDGE('',*,*,#7716,.T.);
#10138=ORIENTED_EDGE('',*,*,#7717,.F.);
#10139=ORIENTED_EDGE('',*,*,#7712,.T.);
#10140=ORIENTED_EDGE('',*,*,#7718,.T.);
#10141=ORIENTED_EDGE('',*,*,#7715,.F.);
#10142=ORIENTED_EDGE('',*,*,#7719,.F.);
#10143=ORIENTED_EDGE('',*,*,#7720,.F.);
#10144=ORIENTED_EDGE('',*,*,#7716,.F.);
#10145=ORIENTED_EDGE('',*,*,#7718,.F.);
#10146=ORIENTED_EDGE('',*,*,#7711,.F.);
#10147=ORIENTED_EDGE('',*,*,#7707,.F.);
#10148=ORIENTED_EDGE('',*,*,#7668,.T.);
#10149=ORIENTED_EDGE('',*,*,#7655,.T.);
#10150=ORIENTED_EDGE('',*,*,#7721,.F.);
#10151=ORIENTED_EDGE('',*,*,#7722,.T.);
#10152=ORIENTED_EDGE('',*,*,#7723,.T.);
#10153=ORIENTED_EDGE('',*,*,#7724,.T.);
#10154=ORIENTED_EDGE('',*,*,#7719,.T.);
#10155=ORIENTED_EDGE('',*,*,#7706,.T.);
#10156=ORIENTED_EDGE('',*,*,#7725,.F.);
#10157=ORIENTED_EDGE('',*,*,#7726,.F.);
#10158=ORIENTED_EDGE('',*,*,#7727,.F.);
#10159=ORIENTED_EDGE('',*,*,#7728,.T.);
#10160=ORIENTED_EDGE('',*,*,#7658,.T.);
#10161=ORIENTED_EDGE('',*,*,#7663,.T.);
#10162=ORIENTED_EDGE('',*,*,#7659,.T.);
#10163=ORIENTED_EDGE('',*,*,#7666,.T.);
#10164=ORIENTED_EDGE('',*,*,#7729,.T.);
#10165=ORIENTED_EDGE('',*,*,#7730,.F.);
#10166=ORIENTED_EDGE('',*,*,#7731,.F.);
#10167=ORIENTED_EDGE('',*,*,#7732,.T.);
#10168=ORIENTED_EDGE('',*,*,#7733,.T.);
#10169=ORIENTED_EDGE('',*,*,#7734,.F.);
#10170=ORIENTED_EDGE('',*,*,#7735,.T.);
#10171=ORIENTED_EDGE('',*,*,#7736,.T.);
#10172=ORIENTED_EDGE('',*,*,#7737,.F.);
#10173=ORIENTED_EDGE('',*,*,#7738,.F.);
#10174=ORIENTED_EDGE('',*,*,#7725,.T.);
#10175=ORIENTED_EDGE('',*,*,#7709,.T.);
#10176=ORIENTED_EDGE('',*,*,#7710,.T.);
#10177=ORIENTED_EDGE('',*,*,#7717,.T.);
#10178=ORIENTED_EDGE('',*,*,#7714,.T.);
#10179=ORIENTED_EDGE('',*,*,#7739,.T.);
#10180=ORIENTED_EDGE('',*,*,#7740,.T.);
#10181=ORIENTED_EDGE('',*,*,#7741,.F.);
#10182=ORIENTED_EDGE('',*,*,#7742,.F.);
#10183=ORIENTED_EDGE('',*,*,#7743,.F.);
#10184=ORIENTED_EDGE('',*,*,#7744,.T.);
#10185=ORIENTED_EDGE('',*,*,#7721,.T.);
#10186=ORIENTED_EDGE('',*,*,#7745,.T.);
#10187=ORIENTED_EDGE('',*,*,#7746,.T.);
#10188=ORIENTED_EDGE('',*,*,#7747,.T.);
#10189=ORIENTED_EDGE('',*,*,#7694,.T.);
#10190=ORIENTED_EDGE('',*,*,#7704,.T.);
#10191=ORIENTED_EDGE('',*,*,#7701,.T.);
#10192=ORIENTED_EDGE('',*,*,#7698,.T.);
#10193=ORIENTED_EDGE('',*,*,#7682,.T.);
#10194=ORIENTED_EDGE('',*,*,#7692,.T.);
#10195=ORIENTED_EDGE('',*,*,#7689,.T.);
#10196=ORIENTED_EDGE('',*,*,#7686,.T.);
#10197=ORIENTED_EDGE('',*,*,#7670,.T.);
#10198=ORIENTED_EDGE('',*,*,#7680,.T.);
#10199=ORIENTED_EDGE('',*,*,#7677,.T.);
#10200=ORIENTED_EDGE('',*,*,#7674,.T.);
#10201=ORIENTED_EDGE('',*,*,#7643,.T.);
#10202=ORIENTED_EDGE('',*,*,#7653,.T.);
#10203=ORIENTED_EDGE('',*,*,#7650,.T.);
#10204=ORIENTED_EDGE('',*,*,#7647,.T.);
#10205=ORIENTED_EDGE('',*,*,#7748,.F.);
#10206=ORIENTED_EDGE('',*,*,#7749,.T.);
#10207=ORIENTED_EDGE('',*,*,#7750,.T.);
#10208=ORIENTED_EDGE('',*,*,#7751,.F.);
#10209=ORIENTED_EDGE('',*,*,#7752,.F.);
#10210=ORIENTED_EDGE('',*,*,#7753,.T.);
#10211=ORIENTED_EDGE('',*,*,#7754,.T.);
#10212=ORIENTED_EDGE('',*,*,#7749,.F.);
#10213=ORIENTED_EDGE('',*,*,#7755,.F.);
#10214=ORIENTED_EDGE('',*,*,#7756,.T.);
#10215=ORIENTED_EDGE('',*,*,#7757,.T.);
#10216=ORIENTED_EDGE('',*,*,#7753,.F.);
#10217=ORIENTED_EDGE('',*,*,#7758,.F.);
#10218=ORIENTED_EDGE('',*,*,#7759,.T.);
#10219=ORIENTED_EDGE('',*,*,#7760,.T.);
#10220=ORIENTED_EDGE('',*,*,#7756,.F.);
#10221=ORIENTED_EDGE('',*,*,#7761,.F.);
#10222=ORIENTED_EDGE('',*,*,#7762,.T.);
#10223=ORIENTED_EDGE('',*,*,#7763,.T.);
#10224=ORIENTED_EDGE('',*,*,#7759,.F.);
#10225=ORIENTED_EDGE('',*,*,#7764,.F.);
#10226=ORIENTED_EDGE('',*,*,#7751,.T.);
#10227=ORIENTED_EDGE('',*,*,#7765,.T.);
#10228=ORIENTED_EDGE('',*,*,#7762,.F.);
#10229=ORIENTED_EDGE('',*,*,#7765,.F.);
#10230=ORIENTED_EDGE('',*,*,#7750,.F.);
#10231=ORIENTED_EDGE('',*,*,#7754,.F.);
#10232=ORIENTED_EDGE('',*,*,#7757,.F.);
#10233=ORIENTED_EDGE('',*,*,#7760,.F.);
#10234=ORIENTED_EDGE('',*,*,#7763,.F.);
#10235=ORIENTED_EDGE('',*,*,#7766,.F.);
#10236=ORIENTED_EDGE('',*,*,#7767,.T.);
#10237=ORIENTED_EDGE('',*,*,#7768,.T.);
#10238=ORIENTED_EDGE('',*,*,#7769,.F.);
#10239=ORIENTED_EDGE('',*,*,#7770,.F.);
#10240=ORIENTED_EDGE('',*,*,#7771,.T.);
#10241=ORIENTED_EDGE('',*,*,#7772,.T.);
#10242=ORIENTED_EDGE('',*,*,#7767,.F.);
#10243=ORIENTED_EDGE('',*,*,#7773,.F.);
#10244=ORIENTED_EDGE('',*,*,#7774,.T.);
#10245=ORIENTED_EDGE('',*,*,#7775,.T.);
#10246=ORIENTED_EDGE('',*,*,#7771,.F.);
#10247=ORIENTED_EDGE('',*,*,#7776,.F.);
#10248=ORIENTED_EDGE('',*,*,#7768,.F.);
#10249=ORIENTED_EDGE('',*,*,#7772,.F.);
#10250=ORIENTED_EDGE('',*,*,#7775,.F.);
#10251=ORIENTED_EDGE('',*,*,#7777,.F.);
#10252=ORIENTED_EDGE('',*,*,#7778,.F.);
#10253=ORIENTED_EDGE('',*,*,#7773,.T.);
#10254=ORIENTED_EDGE('',*,*,#7770,.T.);
#10255=ORIENTED_EDGE('',*,*,#7766,.T.);
#10256=ORIENTED_EDGE('',*,*,#7779,.T.);
#10257=ORIENTED_EDGE('',*,*,#7780,.T.);
#10258=ORIENTED_EDGE('',*,*,#7781,.T.);
#10259=ORIENTED_EDGE('',*,*,#7782,.T.);
#10260=ORIENTED_EDGE('',*,*,#7726,.T.);
#10261=ORIENTED_EDGE('',*,*,#7738,.T.);
#10262=ORIENTED_EDGE('',*,*,#7783,.F.);
#10263=ORIENTED_EDGE('',*,*,#7784,.T.);
#10264=ORIENTED_EDGE('',*,*,#7785,.F.);
#10265=ORIENTED_EDGE('',*,*,#7639,.T.);
#10266=ORIENTED_EDGE('',*,*,#7786,.T.);
#10267=ORIENTED_EDGE('',*,*,#7787,.T.);
#10268=ORIENTED_EDGE('',*,*,#7788,.T.);
#10269=ORIENTED_EDGE('',*,*,#7789,.T.);
#10270=ORIENTED_EDGE('',*,*,#7790,.T.);
#10271=ORIENTED_EDGE('',*,*,#7791,.T.);
#10272=ORIENTED_EDGE('',*,*,#7792,.T.);
#10273=ORIENTED_EDGE('',*,*,#7793,.T.);
#10274=ORIENTED_EDGE('',*,*,#7794,.F.);
#10275=ORIENTED_EDGE('',*,*,#7795,.T.);
#10276=ORIENTED_EDGE('',*,*,#7796,.T.);
#10277=ORIENTED_EDGE('',*,*,#7797,.T.);
#10278=ORIENTED_EDGE('',*,*,#7792,.F.);
#10279=ORIENTED_EDGE('',*,*,#7798,.T.);
#10280=ORIENTED_EDGE('',*,*,#7799,.T.);
#10281=ORIENTED_EDGE('',*,*,#7800,.T.);
#10282=ORIENTED_EDGE('',*,*,#7796,.F.);
#10283=ORIENTED_EDGE('',*,*,#7801,.T.);
#10284=ORIENTED_EDGE('',*,*,#7802,.T.);
#10285=ORIENTED_EDGE('',*,*,#7803,.T.);
#10286=ORIENTED_EDGE('',*,*,#7799,.F.);
#10287=ORIENTED_EDGE('',*,*,#7804,.T.);
#10288=ORIENTED_EDGE('',*,*,#7805,.T.);
#10289=ORIENTED_EDGE('',*,*,#7806,.T.);
#10290=ORIENTED_EDGE('',*,*,#7802,.F.);
#10291=ORIENTED_EDGE('',*,*,#7807,.T.);
#10292=ORIENTED_EDGE('',*,*,#7808,.T.);
#10293=ORIENTED_EDGE('',*,*,#7809,.T.);
#10294=ORIENTED_EDGE('',*,*,#7805,.F.);
#10295=ORIENTED_EDGE('',*,*,#7810,.T.);
#10296=ORIENTED_EDGE('',*,*,#7811,.T.);
#10297=ORIENTED_EDGE('',*,*,#7812,.T.);
#10298=ORIENTED_EDGE('',*,*,#7808,.F.);
#10299=ORIENTED_EDGE('',*,*,#7813,.T.);
#10300=ORIENTED_EDGE('',*,*,#7811,.F.);
#10301=ORIENTED_EDGE('',*,*,#7814,.T.);
#10302=ORIENTED_EDGE('',*,*,#7815,.T.);
#10303=ORIENTED_EDGE('',*,*,#7816,.T.);
#10304=ORIENTED_EDGE('',*,*,#7815,.F.);
#10305=ORIENTED_EDGE('',*,*,#7817,.T.);
#10306=ORIENTED_EDGE('',*,*,#7818,.T.);
#10307=ORIENTED_EDGE('',*,*,#7819,.T.);
#10308=ORIENTED_EDGE('',*,*,#7818,.F.);
#10309=ORIENTED_EDGE('',*,*,#7820,.T.);
#10310=ORIENTED_EDGE('',*,*,#7821,.T.);
#10311=ORIENTED_EDGE('',*,*,#7822,.T.);
#10312=ORIENTED_EDGE('',*,*,#7821,.F.);
#10313=ORIENTED_EDGE('',*,*,#7823,.T.);
#10314=ORIENTED_EDGE('',*,*,#7824,.T.);
#10315=ORIENTED_EDGE('',*,*,#7825,.T.);
#10316=ORIENTED_EDGE('',*,*,#7824,.F.);
#10317=ORIENTED_EDGE('',*,*,#7826,.T.);
#10318=ORIENTED_EDGE('',*,*,#7794,.T.);
#10319=ORIENTED_EDGE('',*,*,#7813,.F.);
#10320=ORIENTED_EDGE('',*,*,#7827,.F.);
#10321=ORIENTED_EDGE('',*,*,#7788,.F.);
#10322=ORIENTED_EDGE('',*,*,#7828,.T.);
#10323=ORIENTED_EDGE('',*,*,#7816,.F.);
#10324=ORIENTED_EDGE('',*,*,#7829,.F.);
#10325=ORIENTED_EDGE('',*,*,#7789,.F.);
#10326=ORIENTED_EDGE('',*,*,#7827,.T.);
#10327=ORIENTED_EDGE('',*,*,#7819,.F.);
#10328=ORIENTED_EDGE('',*,*,#7830,.T.);
#10329=ORIENTED_EDGE('',*,*,#7777,.T.);
#10330=ORIENTED_EDGE('',*,*,#7774,.F.);
#10331=ORIENTED_EDGE('',*,*,#7790,.F.);
#10332=ORIENTED_EDGE('',*,*,#7829,.T.);
#10333=ORIENTED_EDGE('',*,*,#7822,.F.);
#10334=ORIENTED_EDGE('',*,*,#7831,.T.);
#10335=ORIENTED_EDGE('',*,*,#7778,.T.);
#10336=ORIENTED_EDGE('',*,*,#7830,.F.);
#10337=ORIENTED_EDGE('',*,*,#7825,.F.);
#10338=ORIENTED_EDGE('',*,*,#7832,.F.);
#10339=ORIENTED_EDGE('',*,*,#7779,.F.);
#10340=ORIENTED_EDGE('',*,*,#7769,.T.);
#10341=ORIENTED_EDGE('',*,*,#7776,.T.);
#10342=ORIENTED_EDGE('',*,*,#7831,.F.);
#10343=ORIENTED_EDGE('',*,*,#7793,.F.);
#10344=ORIENTED_EDGE('',*,*,#7833,.F.);
#10345=ORIENTED_EDGE('',*,*,#7780,.F.);
#10346=ORIENTED_EDGE('',*,*,#7832,.T.);
#10347=ORIENTED_EDGE('',*,*,#7791,.F.);
#10348=ORIENTED_EDGE('',*,*,#7826,.F.);
#10349=ORIENTED_EDGE('',*,*,#7823,.F.);
#10350=ORIENTED_EDGE('',*,*,#7820,.F.);
#10351=ORIENTED_EDGE('',*,*,#7817,.F.);
#10352=ORIENTED_EDGE('',*,*,#7814,.F.);
#10353=ORIENTED_EDGE('',*,*,#7810,.F.);
#10354=ORIENTED_EDGE('',*,*,#7807,.F.);
#10355=ORIENTED_EDGE('',*,*,#7804,.F.);
#10356=ORIENTED_EDGE('',*,*,#7801,.F.);
#10357=ORIENTED_EDGE('',*,*,#7798,.F.);
#10358=ORIENTED_EDGE('',*,*,#7795,.F.);
#10359=ORIENTED_EDGE('',*,*,#7834,.T.);
#10360=ORIENTED_EDGE('',*,*,#7835,.T.);
#10361=ORIENTED_EDGE('',*,*,#7836,.T.);
#10362=ORIENTED_EDGE('',*,*,#7837,.T.);
#10363=ORIENTED_EDGE('',*,*,#7838,.T.);
#10364=ORIENTED_EDGE('',*,*,#7839,.F.);
#10365=ORIENTED_EDGE('',*,*,#7840,.F.);
#10366=ORIENTED_EDGE('',*,*,#7841,.T.);
#10367=ORIENTED_EDGE('',*,*,#7842,.T.);
#10368=ORIENTED_EDGE('',*,*,#7841,.F.);
#10369=ORIENTED_EDGE('',*,*,#7842,.F.);
#10370=ORIENTED_EDGE('',*,*,#7843,.T.);
#10371=ORIENTED_EDGE('',*,*,#7844,.F.);
#10372=ORIENTED_EDGE('',*,*,#7843,.F.);
#10373=ORIENTED_EDGE('',*,*,#7845,.T.);
#10374=ORIENTED_EDGE('',*,*,#7846,.T.);
#10375=ORIENTED_EDGE('',*,*,#7845,.F.);
#10376=ORIENTED_EDGE('',*,*,#7846,.F.);
#10377=ORIENTED_EDGE('',*,*,#7847,.T.);
#10378=ORIENTED_EDGE('',*,*,#7848,.F.);
#10379=ORIENTED_EDGE('',*,*,#7849,.F.);
#10380=ORIENTED_EDGE('',*,*,#7850,.T.);
#10381=ORIENTED_EDGE('',*,*,#7851,.T.);
#10382=ORIENTED_EDGE('',*,*,#7850,.F.);
#10383=ORIENTED_EDGE('',*,*,#7852,.F.);
#10384=ORIENTED_EDGE('',*,*,#7847,.F.);
#10385=ORIENTED_EDGE('',*,*,#7851,.F.);
#10386=ORIENTED_EDGE('',*,*,#7853,.T.);
#10387=ORIENTED_EDGE('',*,*,#7854,.F.);
#10388=ORIENTED_EDGE('',*,*,#7855,.F.);
#10389=ORIENTED_EDGE('',*,*,#7856,.F.);
#10390=ORIENTED_EDGE('',*,*,#7853,.F.);
#10391=ORIENTED_EDGE('',*,*,#7854,.T.);
#10392=ORIENTED_EDGE('',*,*,#7856,.T.);
#10393=ORIENTED_EDGE('',*,*,#7857,.F.);
#10394=ORIENTED_EDGE('',*,*,#7858,.F.);
#10395=ORIENTED_EDGE('',*,*,#7859,.F.);
#10396=ORIENTED_EDGE('',*,*,#7860,.T.);
#10397=ORIENTED_EDGE('',*,*,#7861,.T.);
#10398=ORIENTED_EDGE('',*,*,#7862,.F.);
#10399=ORIENTED_EDGE('',*,*,#7863,.T.);
#10400=ORIENTED_EDGE('',*,*,#7864,.T.);
#10401=ORIENTED_EDGE('',*,*,#7865,.F.);
#10402=ORIENTED_EDGE('',*,*,#7784,.F.);
#10403=ORIENTED_EDGE('',*,*,#7866,.F.);
#10404=ORIENTED_EDGE('',*,*,#7867,.T.);
#10405=ORIENTED_EDGE('',*,*,#7868,.T.);
#10406=ORIENTED_EDGE('',*,*,#7869,.F.);
#10407=ORIENTED_EDGE('',*,*,#7844,.T.);
#10408=ORIENTED_EDGE('',*,*,#7870,.T.);
#10409=ORIENTED_EDGE('',*,*,#7871,.T.);
#10410=ORIENTED_EDGE('',*,*,#7872,.T.);
#10411=ORIENTED_EDGE('',*,*,#7873,.T.);
#10412=ORIENTED_EDGE('',*,*,#7874,.T.);
#10413=ORIENTED_EDGE('',*,*,#7875,.T.);
#10414=ORIENTED_EDGE('',*,*,#7876,.T.);
#10415=ORIENTED_EDGE('',*,*,#7877,.T.);
#10416=ORIENTED_EDGE('',*,*,#7878,.T.);
#10417=ORIENTED_EDGE('',*,*,#7879,.T.);
#10418=ORIENTED_EDGE('',*,*,#7880,.T.);
#10419=ORIENTED_EDGE('',*,*,#7881,.T.);
#10420=ORIENTED_EDGE('',*,*,#7882,.T.);
#10421=ORIENTED_EDGE('',*,*,#7883,.T.);
#10422=ORIENTED_EDGE('',*,*,#7884,.T.);
#10423=ORIENTED_EDGE('',*,*,#7885,.T.);
#10424=ORIENTED_EDGE('',*,*,#7886,.T.);
#10425=ORIENTED_EDGE('',*,*,#7887,.T.);
#10426=ORIENTED_EDGE('',*,*,#7888,.T.);
#10427=ORIENTED_EDGE('',*,*,#7889,.T.);
#10428=ORIENTED_EDGE('',*,*,#7890,.T.);
#10429=ORIENTED_EDGE('',*,*,#7891,.T.);
#10430=ORIENTED_EDGE('',*,*,#7892,.T.);
#10431=ORIENTED_EDGE('',*,*,#7893,.T.);
#10432=ORIENTED_EDGE('',*,*,#7894,.T.);
#10433=ORIENTED_EDGE('',*,*,#7895,.T.);
#10434=ORIENTED_EDGE('',*,*,#7894,.F.);
#10435=ORIENTED_EDGE('',*,*,#7895,.F.);
#10436=ORIENTED_EDGE('',*,*,#7896,.T.);
#10437=ORIENTED_EDGE('',*,*,#7897,.T.);
#10438=ORIENTED_EDGE('',*,*,#7896,.F.);
#10439=ORIENTED_EDGE('',*,*,#7898,.F.);
#10440=ORIENTED_EDGE('',*,*,#7899,.F.);
#10441=ORIENTED_EDGE('',*,*,#7897,.F.);
#10442=ORIENTED_EDGE('',*,*,#7900,.T.);
#10443=ORIENTED_EDGE('',*,*,#7867,.F.);
#10444=ORIENTED_EDGE('',*,*,#7901,.F.);
#10445=ORIENTED_EDGE('',*,*,#7868,.F.);
#10446=ORIENTED_EDGE('',*,*,#7900,.F.);
#10447=ORIENTED_EDGE('',*,*,#7855,.T.);
#10448=ORIENTED_EDGE('',*,*,#7869,.T.);
#10449=ORIENTED_EDGE('',*,*,#7901,.T.);
#10450=ORIENTED_EDGE('',*,*,#7866,.T.);
#10451=ORIENTED_EDGE('',*,*,#7783,.T.);
#10452=ORIENTED_EDGE('',*,*,#7737,.T.);
#10453=ORIENTED_EDGE('',*,*,#7902,.T.);
#10454=ORIENTED_EDGE('',*,*,#7734,.T.);
#10455=ORIENTED_EDGE('',*,*,#7903,.T.);
#10456=ORIENTED_EDGE('',*,*,#7731,.T.);
#10457=ORIENTED_EDGE('',*,*,#7904,.T.);
#10458=ORIENTED_EDGE('',*,*,#7857,.T.);
#10459=ORIENTED_EDGE('',*,*,#7905,.T.);
#10460=ORIENTED_EDGE('',*,*,#7906,.T.);
#10461=ORIENTED_EDGE('',*,*,#7905,.F.);
#10462=ORIENTED_EDGE('',*,*,#7906,.F.);
#10463=ORIENTED_EDGE('',*,*,#7907,.T.);
#10464=ORIENTED_EDGE('',*,*,#7908,.T.);
#10465=ORIENTED_EDGE('',*,*,#7907,.F.);
#10466=ORIENTED_EDGE('',*,*,#7908,.F.);
#10467=ORIENTED_EDGE('',*,*,#7909,.T.);
#10468=ORIENTED_EDGE('',*,*,#7860,.F.);
#10469=ORIENTED_EDGE('',*,*,#7910,.F.);
#10470=ORIENTED_EDGE('',*,*,#7861,.F.);
#10471=ORIENTED_EDGE('',*,*,#7909,.F.);
#10472=ORIENTED_EDGE('',*,*,#7910,.T.);
#10473=ORIENTED_EDGE('',*,*,#7859,.T.);
#10474=ORIENTED_EDGE('',*,*,#7911,.T.);
#10475=ORIENTED_EDGE('',*,*,#7640,.T.);
#10476=ORIENTED_EDGE('',*,*,#7785,.T.);
#10477=ORIENTED_EDGE('',*,*,#7865,.T.);
#10478=ORIENTED_EDGE('',*,*,#7912,.T.);
#10479=ORIENTED_EDGE('',*,*,#7862,.T.);
#10480=ORIENTED_EDGE('',*,*,#7913,.T.);
#10481=ORIENTED_EDGE('',*,*,#7914,.T.);
#10482=ORIENTED_EDGE('',*,*,#7913,.F.);
#10483=ORIENTED_EDGE('',*,*,#7914,.F.);
#10484=ORIENTED_EDGE('',*,*,#7915,.T.);
#10485=ORIENTED_EDGE('',*,*,#7916,.T.);
#10486=ORIENTED_EDGE('',*,*,#7915,.F.);
#10487=ORIENTED_EDGE('',*,*,#7916,.F.);
#10488=ORIENTED_EDGE('',*,*,#7917,.T.);
#10489=ORIENTED_EDGE('',*,*,#7863,.F.);
#10490=ORIENTED_EDGE('',*,*,#7912,.F.);
#10491=ORIENTED_EDGE('',*,*,#7864,.F.);
#10492=ORIENTED_EDGE('',*,*,#7917,.F.);
#10493=ORIENTED_EDGE('',*,*,#7918,.T.);
#10494=ORIENTED_EDGE('',*,*,#7919,.T.);
#10495=ORIENTED_EDGE('',*,*,#7918,.F.);
#10496=ORIENTED_EDGE('',*,*,#7919,.F.);
#10497=ORIENTED_EDGE('',*,*,#7920,.T.);
#10498=ORIENTED_EDGE('',*,*,#7921,.T.);
#10499=ORIENTED_EDGE('',*,*,#7920,.F.);
#10500=ORIENTED_EDGE('',*,*,#7921,.F.);
#10501=ORIENTED_EDGE('',*,*,#7922,.T.);
#10502=ORIENTED_EDGE('',*,*,#7838,.F.);
#10503=ORIENTED_EDGE('',*,*,#7922,.F.);
#10504=ORIENTED_EDGE('',*,*,#7923,.T.);
#10505=ORIENTED_EDGE('',*,*,#7924,.T.);
#10506=ORIENTED_EDGE('',*,*,#7923,.F.);
#10507=ORIENTED_EDGE('',*,*,#7924,.F.);
#10508=ORIENTED_EDGE('',*,*,#7925,.T.);
#10509=ORIENTED_EDGE('',*,*,#7926,.T.);
#10510=ORIENTED_EDGE('',*,*,#7925,.F.);
#10511=ORIENTED_EDGE('',*,*,#7926,.F.);
#10512=ORIENTED_EDGE('',*,*,#7927,.T.);
#10513=ORIENTED_EDGE('',*,*,#7928,.F.);
#10514=ORIENTED_EDGE('',*,*,#7927,.F.);
#10515=ORIENTED_EDGE('',*,*,#7929,.T.);
#10516=ORIENTED_EDGE('',*,*,#7930,.T.);
#10517=ORIENTED_EDGE('',*,*,#7929,.F.);
#10518=ORIENTED_EDGE('',*,*,#7930,.F.);
#10519=ORIENTED_EDGE('',*,*,#7931,.T.);
#10520=ORIENTED_EDGE('',*,*,#7932,.T.);
#10521=ORIENTED_EDGE('',*,*,#7931,.F.);
#10522=ORIENTED_EDGE('',*,*,#7932,.F.);
#10523=ORIENTED_EDGE('',*,*,#7933,.T.);
#10524=ORIENTED_EDGE('',*,*,#7837,.F.);
#10525=ORIENTED_EDGE('',*,*,#7933,.F.);
#10526=ORIENTED_EDGE('',*,*,#7934,.T.);
#10527=ORIENTED_EDGE('',*,*,#7935,.T.);
#10528=ORIENTED_EDGE('',*,*,#7934,.F.);
#10529=ORIENTED_EDGE('',*,*,#7935,.F.);
#10530=ORIENTED_EDGE('',*,*,#7936,.T.);
#10531=ORIENTED_EDGE('',*,*,#7937,.T.);
#10532=ORIENTED_EDGE('',*,*,#7936,.F.);
#10533=ORIENTED_EDGE('',*,*,#7937,.F.);
#10534=ORIENTED_EDGE('',*,*,#7938,.T.);
#10535=ORIENTED_EDGE('',*,*,#7939,.F.);
#10536=ORIENTED_EDGE('',*,*,#7938,.F.);
#10537=ORIENTED_EDGE('',*,*,#7940,.T.);
#10538=ORIENTED_EDGE('',*,*,#7941,.T.);
#10539=ORIENTED_EDGE('',*,*,#7940,.F.);
#10540=ORIENTED_EDGE('',*,*,#7941,.F.);
#10541=ORIENTED_EDGE('',*,*,#7942,.T.);
#10542=ORIENTED_EDGE('',*,*,#7943,.T.);
#10543=ORIENTED_EDGE('',*,*,#7942,.F.);
#10544=ORIENTED_EDGE('',*,*,#7943,.F.);
#10545=ORIENTED_EDGE('',*,*,#7944,.T.);
#10546=ORIENTED_EDGE('',*,*,#7836,.F.);
#10547=ORIENTED_EDGE('',*,*,#7944,.F.);
#10548=ORIENTED_EDGE('',*,*,#7945,.T.);
#10549=ORIENTED_EDGE('',*,*,#7946,.T.);
#10550=ORIENTED_EDGE('',*,*,#7945,.F.);
#10551=ORIENTED_EDGE('',*,*,#7946,.F.);
#10552=ORIENTED_EDGE('',*,*,#7947,.T.);
#10553=ORIENTED_EDGE('',*,*,#7948,.T.);
#10554=ORIENTED_EDGE('',*,*,#7947,.F.);
#10555=ORIENTED_EDGE('',*,*,#7948,.F.);
#10556=ORIENTED_EDGE('',*,*,#7949,.T.);
#10557=ORIENTED_EDGE('',*,*,#7950,.F.);
#10558=ORIENTED_EDGE('',*,*,#7949,.F.);
#10559=ORIENTED_EDGE('',*,*,#7951,.T.);
#10560=ORIENTED_EDGE('',*,*,#7952,.T.);
#10561=ORIENTED_EDGE('',*,*,#7951,.F.);
#10562=ORIENTED_EDGE('',*,*,#7952,.F.);
#10563=ORIENTED_EDGE('',*,*,#7953,.T.);
#10564=ORIENTED_EDGE('',*,*,#7954,.T.);
#10565=ORIENTED_EDGE('',*,*,#7953,.F.);
#10566=ORIENTED_EDGE('',*,*,#7954,.F.);
#10567=ORIENTED_EDGE('',*,*,#7955,.T.);
#10568=ORIENTED_EDGE('',*,*,#7835,.F.);
#10569=ORIENTED_EDGE('',*,*,#7955,.F.);
#10570=ORIENTED_EDGE('',*,*,#7956,.T.);
#10571=ORIENTED_EDGE('',*,*,#7957,.T.);
#10572=ORIENTED_EDGE('',*,*,#7956,.F.);
#10573=ORIENTED_EDGE('',*,*,#7957,.F.);
#10574=ORIENTED_EDGE('',*,*,#7958,.T.);
#10575=ORIENTED_EDGE('',*,*,#7959,.T.);
#10576=ORIENTED_EDGE('',*,*,#7958,.F.);
#10577=ORIENTED_EDGE('',*,*,#7959,.F.);
#10578=ORIENTED_EDGE('',*,*,#7960,.T.);
#10579=ORIENTED_EDGE('',*,*,#7961,.F.);
#10580=ORIENTED_EDGE('',*,*,#7960,.F.);
#10581=ORIENTED_EDGE('',*,*,#7962,.T.);
#10582=ORIENTED_EDGE('',*,*,#7963,.T.);
#10583=ORIENTED_EDGE('',*,*,#7962,.F.);
#10584=ORIENTED_EDGE('',*,*,#7963,.F.);
#10585=ORIENTED_EDGE('',*,*,#7964,.T.);
#10586=ORIENTED_EDGE('',*,*,#7965,.T.);
#10587=ORIENTED_EDGE('',*,*,#7964,.F.);
#10588=ORIENTED_EDGE('',*,*,#7965,.F.);
#10589=ORIENTED_EDGE('',*,*,#7966,.T.);
#10590=ORIENTED_EDGE('',*,*,#7747,.F.);
#10591=ORIENTED_EDGE('',*,*,#7966,.F.);
#10592=ORIENTED_EDGE('',*,*,#7967,.T.);
#10593=ORIENTED_EDGE('',*,*,#7968,.T.);
#10594=ORIENTED_EDGE('',*,*,#7967,.F.);
#10595=ORIENTED_EDGE('',*,*,#7968,.F.);
#10596=ORIENTED_EDGE('',*,*,#7969,.T.);
#10597=ORIENTED_EDGE('',*,*,#7970,.T.);
#10598=ORIENTED_EDGE('',*,*,#7969,.F.);
#10599=ORIENTED_EDGE('',*,*,#7970,.F.);
#10600=ORIENTED_EDGE('',*,*,#7971,.T.);
#10601=ORIENTED_EDGE('',*,*,#7746,.F.);
#10602=ORIENTED_EDGE('',*,*,#7971,.F.);
#10603=ORIENTED_EDGE('',*,*,#7972,.T.);
#10604=ORIENTED_EDGE('',*,*,#7973,.T.);
#10605=ORIENTED_EDGE('',*,*,#7972,.F.);
#10606=ORIENTED_EDGE('',*,*,#7973,.F.);
#10607=ORIENTED_EDGE('',*,*,#7974,.T.);
#10608=ORIENTED_EDGE('',*,*,#7975,.T.);
#10609=ORIENTED_EDGE('',*,*,#7974,.F.);
#10610=ORIENTED_EDGE('',*,*,#7848,.T.);
#10611=ORIENTED_EDGE('',*,*,#7852,.T.);
#10612=ORIENTED_EDGE('',*,*,#7849,.T.);
#10613=ORIENTED_EDGE('',*,*,#7975,.F.);
#10614=ORIENTED_EDGE('',*,*,#7976,.T.);
#10615=ORIENTED_EDGE('',*,*,#7732,.F.);
#10616=ORIENTED_EDGE('',*,*,#7903,.F.);
#10617=ORIENTED_EDGE('',*,*,#7733,.F.);
#10618=ORIENTED_EDGE('',*,*,#7976,.F.);
#10619=ORIENTED_EDGE('',*,*,#7977,.T.);
#10620=ORIENTED_EDGE('',*,*,#7978,.T.);
#10621=ORIENTED_EDGE('',*,*,#7977,.F.);
#10622=ORIENTED_EDGE('',*,*,#7978,.F.);
#10623=ORIENTED_EDGE('',*,*,#7979,.T.);
#10624=ORIENTED_EDGE('',*,*,#7898,.T.);
#10625=ORIENTED_EDGE('',*,*,#7980,.T.);
#10626=ORIENTED_EDGE('',*,*,#7981,.T.);
#10627=ORIENTED_EDGE('',*,*,#7980,.F.);
#10628=ORIENTED_EDGE('',*,*,#7899,.T.);
#10629=ORIENTED_EDGE('',*,*,#7979,.F.);
#10630=ORIENTED_EDGE('',*,*,#7981,.F.);
#10631=ORIENTED_EDGE('',*,*,#7982,.T.);
#10632=ORIENTED_EDGE('',*,*,#7735,.F.);
#10633=ORIENTED_EDGE('',*,*,#7902,.F.);
#10634=ORIENTED_EDGE('',*,*,#7736,.F.);
#10635=ORIENTED_EDGE('',*,*,#7982,.F.);
#10636=ORIENTED_EDGE('',*,*,#7983,.F.);
#10637=ORIENTED_EDGE('',*,*,#7984,.T.);
#10638=ORIENTED_EDGE('',*,*,#7985,.T.);
#10639=ORIENTED_EDGE('',*,*,#7984,.F.);
#10640=ORIENTED_EDGE('',*,*,#7985,.F.);
#10641=ORIENTED_EDGE('',*,*,#7986,.T.);
#10642=ORIENTED_EDGE('',*,*,#7987,.F.);
#10643=ORIENTED_EDGE('',*,*,#7986,.F.);
#10644=ORIENTED_EDGE('',*,*,#7988,.F.);
#10645=ORIENTED_EDGE('',*,*,#7989,.T.);
#10646=ORIENTED_EDGE('',*,*,#7990,.T.);
#10647=ORIENTED_EDGE('',*,*,#7989,.F.);
#10648=ORIENTED_EDGE('',*,*,#7990,.F.);
#10649=ORIENTED_EDGE('',*,*,#7991,.T.);
#10650=ORIENTED_EDGE('',*,*,#7992,.F.);
#10651=ORIENTED_EDGE('',*,*,#7991,.F.);
#10652=ORIENTED_EDGE('',*,*,#7993,.F.);
#10653=ORIENTED_EDGE('',*,*,#7994,.T.);
#10654=ORIENTED_EDGE('',*,*,#7995,.T.);
#10655=ORIENTED_EDGE('',*,*,#7994,.F.);
#10656=ORIENTED_EDGE('',*,*,#7995,.F.);
#10657=ORIENTED_EDGE('',*,*,#7996,.T.);
#10658=ORIENTED_EDGE('',*,*,#7997,.F.);
#10659=ORIENTED_EDGE('',*,*,#7996,.F.);
#10660=ORIENTED_EDGE('',*,*,#7998,.F.);
#10661=ORIENTED_EDGE('',*,*,#7999,.T.);
#10662=ORIENTED_EDGE('',*,*,#8000,.T.);
#10663=ORIENTED_EDGE('',*,*,#7999,.F.);
#10664=ORIENTED_EDGE('',*,*,#8000,.F.);
#10665=ORIENTED_EDGE('',*,*,#8001,.T.);
#10666=ORIENTED_EDGE('',*,*,#8002,.F.);
#10667=ORIENTED_EDGE('',*,*,#8001,.F.);
#10668=ORIENTED_EDGE('',*,*,#8003,.F.);
#10669=ORIENTED_EDGE('',*,*,#8004,.F.);
#10670=ORIENTED_EDGE('',*,*,#7626,.F.);
#10671=ORIENTED_EDGE('',*,*,#7631,.T.);
#10672=ORIENTED_EDGE('',*,*,#8005,.F.);
#10673=ORIENTED_EDGE('',*,*,#7632,.F.);
#10674=ORIENTED_EDGE('',*,*,#7627,.F.);
#10675=ORIENTED_EDGE('',*,*,#8004,.T.);
#10676=ORIENTED_EDGE('',*,*,#7993,.T.);
#10677=ORIENTED_EDGE('',*,*,#7669,.T.);
#10678=ORIENTED_EDGE('',*,*,#7724,.F.);
#10679=ORIENTED_EDGE('',*,*,#8006,.T.);
#10680=ORIENTED_EDGE('',*,*,#8007,.F.);
#10681=ORIENTED_EDGE('',*,*,#7729,.F.);
#10682=ORIENTED_EDGE('',*,*,#7665,.T.);
#10683=ORIENTED_EDGE('',*,*,#8008,.F.);
#10684=ORIENTED_EDGE('',*,*,#8006,.F.);
#10685=ORIENTED_EDGE('',*,*,#7723,.F.);
#10686=ORIENTED_EDGE('',*,*,#8009,.T.);
#10687=ORIENTED_EDGE('',*,*,#7744,.F.);
#10688=ORIENTED_EDGE('',*,*,#8010,.F.);
#10689=ORIENTED_EDGE('',*,*,#8009,.F.);
#10690=ORIENTED_EDGE('',*,*,#7722,.F.);
#10691=ORIENTED_EDGE('',*,*,#7983,.T.);
#10692=ORIENTED_EDGE('',*,*,#8005,.T.);
#10693=ORIENTED_EDGE('',*,*,#8003,.T.);
#10694=ORIENTED_EDGE('',*,*,#7630,.T.);
#10695=ORIENTED_EDGE('',*,*,#7641,.T.);
#10696=ORIENTED_EDGE('',*,*,#7911,.F.);
#10697=ORIENTED_EDGE('',*,*,#7858,.T.);
#10698=ORIENTED_EDGE('',*,*,#7904,.F.);
#10699=ORIENTED_EDGE('',*,*,#7730,.T.);
#10700=ORIENTED_EDGE('',*,*,#8007,.T.);
#10701=ORIENTED_EDGE('',*,*,#8008,.T.);
#10702=ORIENTED_EDGE('',*,*,#8010,.T.);
#10703=ORIENTED_EDGE('',*,*,#7743,.T.);
#10704=ORIENTED_EDGE('',*,*,#8011,.F.);
#10705=ORIENTED_EDGE('',*,*,#8012,.T.);
#10706=ORIENTED_EDGE('',*,*,#8013,.T.);
#10707=ORIENTED_EDGE('',*,*,#8014,.T.);
#10708=ORIENTED_EDGE('',*,*,#8015,.T.);
#10709=ORIENTED_EDGE('',*,*,#8016,.T.);
#10710=ORIENTED_EDGE('',*,*,#8017,.F.);
#10711=ORIENTED_EDGE('',*,*,#7633,.T.);
#10712=ORIENTED_EDGE('',*,*,#7748,.T.);
#10713=ORIENTED_EDGE('',*,*,#7764,.T.);
#10714=ORIENTED_EDGE('',*,*,#7761,.T.);
#10715=ORIENTED_EDGE('',*,*,#7758,.T.);
#10716=ORIENTED_EDGE('',*,*,#7755,.T.);
#10717=ORIENTED_EDGE('',*,*,#7752,.T.);
#10718=ORIENTED_EDGE('',*,*,#7928,.T.);
#10719=ORIENTED_EDGE('',*,*,#7939,.T.);
#10720=ORIENTED_EDGE('',*,*,#7950,.T.);
#10721=ORIENTED_EDGE('',*,*,#7961,.T.);
#10722=ORIENTED_EDGE('',*,*,#8018,.T.);
#10723=ORIENTED_EDGE('',*,*,#8019,.F.);
#10724=ORIENTED_EDGE('',*,*,#8020,.F.);
#10725=ORIENTED_EDGE('',*,*,#8021,.T.);
#10726=ORIENTED_EDGE('',*,*,#7636,.F.);
#10727=ORIENTED_EDGE('',*,*,#7998,.T.);
#10728=ORIENTED_EDGE('',*,*,#7610,.T.);
#10729=ORIENTED_EDGE('',*,*,#7637,.F.);
#10730=ORIENTED_EDGE('',*,*,#8021,.F.);
#10731=ORIENTED_EDGE('',*,*,#8022,.F.);
#10732=ORIENTED_EDGE('',*,*,#8023,.F.);
#10733=ORIENTED_EDGE('',*,*,#7623,.T.);
#10734=ORIENTED_EDGE('',*,*,#7812,.F.);
#10735=ORIENTED_EDGE('',*,*,#7828,.F.);
#10736=ORIENTED_EDGE('',*,*,#7787,.F.);
#10737=ORIENTED_EDGE('',*,*,#8024,.F.);
#10738=ORIENTED_EDGE('',*,*,#8022,.T.);
#10739=ORIENTED_EDGE('',*,*,#8020,.T.);
#10740=ORIENTED_EDGE('',*,*,#8025,.F.);
#10741=ORIENTED_EDGE('',*,*,#8026,.F.);
#10742=ORIENTED_EDGE('',*,*,#7624,.T.);
#10743=ORIENTED_EDGE('',*,*,#8023,.T.);
#10744=ORIENTED_EDGE('',*,*,#8024,.T.);
#10745=ORIENTED_EDGE('',*,*,#7786,.F.);
#10746=ORIENTED_EDGE('',*,*,#7638,.F.);
#10747=ORIENTED_EDGE('',*,*,#7614,.T.);
#10748=ORIENTED_EDGE('',*,*,#7800,.F.);
#10749=ORIENTED_EDGE('',*,*,#8027,.F.);
#10750=ORIENTED_EDGE('',*,*,#8028,.F.);
#10751=ORIENTED_EDGE('',*,*,#8029,.F.);
#10752=ORIENTED_EDGE('',*,*,#8030,.T.);
#10753=ORIENTED_EDGE('',*,*,#7727,.T.);
#10754=ORIENTED_EDGE('',*,*,#7782,.F.);
#10755=ORIENTED_EDGE('',*,*,#8031,.F.);
#10756=ORIENTED_EDGE('',*,*,#8032,.F.);
#10757=ORIENTED_EDGE('',*,*,#7740,.F.);
#10758=ORIENTED_EDGE('',*,*,#8033,.T.);
#10759=ORIENTED_EDGE('',*,*,#8029,.T.);
#10760=ORIENTED_EDGE('',*,*,#7988,.T.);
#10761=ORIENTED_EDGE('',*,*,#7720,.T.);
#10762=ORIENTED_EDGE('',*,*,#7728,.F.);
#10763=ORIENTED_EDGE('',*,*,#8030,.F.);
#10764=ORIENTED_EDGE('',*,*,#8033,.F.);
#10765=ORIENTED_EDGE('',*,*,#7739,.F.);
#10766=ORIENTED_EDGE('',*,*,#7713,.T.);
#10767=ORIENTED_EDGE('',*,*,#7809,.F.);
#10768=ORIENTED_EDGE('',*,*,#8026,.T.);
#10769=ORIENTED_EDGE('',*,*,#8034,.F.);
#10770=ORIENTED_EDGE('',*,*,#8035,.T.);
#10771=ORIENTED_EDGE('',*,*,#7797,.F.);
#10772=ORIENTED_EDGE('',*,*,#8031,.T.);
#10773=ORIENTED_EDGE('',*,*,#7781,.F.);
#10774=ORIENTED_EDGE('',*,*,#7833,.T.);
#10775=ORIENTED_EDGE('',*,*,#7803,.F.);
#10776=ORIENTED_EDGE('',*,*,#8036,.F.);
#10777=ORIENTED_EDGE('',*,*,#8037,.F.);
#10778=ORIENTED_EDGE('',*,*,#8027,.T.);
#10779=ORIENTED_EDGE('',*,*,#8025,.T.);
#10780=ORIENTED_EDGE('',*,*,#8019,.T.);
#10781=ORIENTED_EDGE('',*,*,#7635,.T.);
#10782=ORIENTED_EDGE('',*,*,#8038,.F.);
#10783=ORIENTED_EDGE('',*,*,#8039,.T.);
#10784=ORIENTED_EDGE('',*,*,#8040,.T.);
#10785=ORIENTED_EDGE('',*,*,#8041,.T.);
#10786=ORIENTED_EDGE('',*,*,#8042,.T.);
#10787=ORIENTED_EDGE('',*,*,#8043,.T.);
#10788=ORIENTED_EDGE('',*,*,#8044,.F.);
#10789=ORIENTED_EDGE('',*,*,#7741,.T.);
#10790=ORIENTED_EDGE('',*,*,#8032,.T.);
#10791=ORIENTED_EDGE('',*,*,#8028,.T.);
#10792=ORIENTED_EDGE('',*,*,#8037,.T.);
#10793=ORIENTED_EDGE('',*,*,#8045,.T.);
#10794=ORIENTED_EDGE('',*,*,#8034,.T.);
#10795=ORIENTED_EDGE('',*,*,#8042,.F.);
#10796=ORIENTED_EDGE('',*,*,#8046,.T.);
#10797=ORIENTED_EDGE('',*,*,#8013,.F.);
#10798=ORIENTED_EDGE('',*,*,#8047,.F.);
#10799=ORIENTED_EDGE('',*,*,#8040,.F.);
#10800=ORIENTED_EDGE('',*,*,#8048,.F.);
#10801=ORIENTED_EDGE('',*,*,#8015,.F.);
#10802=ORIENTED_EDGE('',*,*,#8049,.T.);
#10803=ORIENTED_EDGE('',*,*,#8041,.F.);
#10804=ORIENTED_EDGE('',*,*,#8049,.F.);
#10805=ORIENTED_EDGE('',*,*,#8014,.F.);
#10806=ORIENTED_EDGE('',*,*,#8046,.F.);
#10807=ORIENTED_EDGE('',*,*,#8048,.T.);
#10808=ORIENTED_EDGE('',*,*,#8039,.F.);
#10809=ORIENTED_EDGE('',*,*,#8050,.F.);
#10810=ORIENTED_EDGE('',*,*,#8016,.F.);
#10811=ORIENTED_EDGE('',*,*,#7997,.T.);
#10812=ORIENTED_EDGE('',*,*,#8002,.T.);
#10813=ORIENTED_EDGE('',*,*,#8047,.T.);
#10814=ORIENTED_EDGE('',*,*,#8012,.F.);
#10815=ORIENTED_EDGE('',*,*,#8051,.F.);
#10816=ORIENTED_EDGE('',*,*,#8043,.F.);
#10817=ORIENTED_EDGE('',*,*,#7987,.T.);
#10818=ORIENTED_EDGE('',*,*,#7992,.T.);
#10819=ORIENTED_EDGE('',*,*,#7890,.F.);
#10820=ORIENTED_EDGE('',*,*,#8052,.T.);
#10821=ORIENTED_EDGE('',*,*,#8053,.T.);
#10822=ORIENTED_EDGE('',*,*,#8054,.F.);
#10823=ORIENTED_EDGE('',*,*,#7893,.F.);
#10824=ORIENTED_EDGE('',*,*,#8055,.T.);
#10825=ORIENTED_EDGE('',*,*,#8056,.T.);
#10826=ORIENTED_EDGE('',*,*,#8052,.F.);
#10827=ORIENTED_EDGE('',*,*,#7892,.F.);
#10828=ORIENTED_EDGE('',*,*,#8057,.T.);
#10829=ORIENTED_EDGE('',*,*,#8058,.T.);
#10830=ORIENTED_EDGE('',*,*,#8055,.F.);
#10831=ORIENTED_EDGE('',*,*,#7891,.F.);
#10832=ORIENTED_EDGE('',*,*,#8054,.T.);
#10833=ORIENTED_EDGE('',*,*,#8059,.T.);
#10834=ORIENTED_EDGE('',*,*,#8057,.F.);
#10835=ORIENTED_EDGE('',*,*,#8059,.F.);
#10836=ORIENTED_EDGE('',*,*,#8053,.F.);
#10837=ORIENTED_EDGE('',*,*,#8056,.F.);
#10838=ORIENTED_EDGE('',*,*,#8058,.F.);
#10839=ORIENTED_EDGE('',*,*,#7886,.F.);
#10840=ORIENTED_EDGE('',*,*,#8060,.T.);
#10841=ORIENTED_EDGE('',*,*,#8061,.T.);
#10842=ORIENTED_EDGE('',*,*,#8062,.F.);
#10843=ORIENTED_EDGE('',*,*,#7889,.F.);
#10844=ORIENTED_EDGE('',*,*,#8063,.T.);
#10845=ORIENTED_EDGE('',*,*,#8064,.T.);
#10846=ORIENTED_EDGE('',*,*,#8060,.F.);
#10847=ORIENTED_EDGE('',*,*,#7888,.F.);
#10848=ORIENTED_EDGE('',*,*,#8065,.T.);
#10849=ORIENTED_EDGE('',*,*,#8066,.T.);
#10850=ORIENTED_EDGE('',*,*,#8063,.F.);
#10851=ORIENTED_EDGE('',*,*,#7887,.F.);
#10852=ORIENTED_EDGE('',*,*,#8062,.T.);
#10853=ORIENTED_EDGE('',*,*,#8067,.T.);
#10854=ORIENTED_EDGE('',*,*,#8065,.F.);
#10855=ORIENTED_EDGE('',*,*,#8067,.F.);
#10856=ORIENTED_EDGE('',*,*,#8061,.F.);
#10857=ORIENTED_EDGE('',*,*,#8064,.F.);
#10858=ORIENTED_EDGE('',*,*,#8066,.F.);
#10859=ORIENTED_EDGE('',*,*,#7882,.F.);
#10860=ORIENTED_EDGE('',*,*,#8068,.T.);
#10861=ORIENTED_EDGE('',*,*,#8069,.T.);
#10862=ORIENTED_EDGE('',*,*,#8070,.F.);
#10863=ORIENTED_EDGE('',*,*,#7885,.F.);
#10864=ORIENTED_EDGE('',*,*,#8071,.T.);
#10865=ORIENTED_EDGE('',*,*,#8072,.T.);
#10866=ORIENTED_EDGE('',*,*,#8068,.F.);
#10867=ORIENTED_EDGE('',*,*,#7884,.F.);
#10868=ORIENTED_EDGE('',*,*,#8073,.T.);
#10869=ORIENTED_EDGE('',*,*,#8074,.T.);
#10870=ORIENTED_EDGE('',*,*,#8071,.F.);
#10871=ORIENTED_EDGE('',*,*,#7883,.F.);
#10872=ORIENTED_EDGE('',*,*,#8070,.T.);
#10873=ORIENTED_EDGE('',*,*,#8075,.T.);
#10874=ORIENTED_EDGE('',*,*,#8073,.F.);
#10875=ORIENTED_EDGE('',*,*,#8075,.F.);
#10876=ORIENTED_EDGE('',*,*,#8069,.F.);
#10877=ORIENTED_EDGE('',*,*,#8072,.F.);
#10878=ORIENTED_EDGE('',*,*,#8074,.F.);
#10879=ORIENTED_EDGE('',*,*,#7878,.F.);
#10880=ORIENTED_EDGE('',*,*,#8076,.T.);
#10881=ORIENTED_EDGE('',*,*,#8077,.T.);
#10882=ORIENTED_EDGE('',*,*,#8078,.F.);
#10883=ORIENTED_EDGE('',*,*,#7881,.F.);
#10884=ORIENTED_EDGE('',*,*,#8079,.T.);
#10885=ORIENTED_EDGE('',*,*,#8080,.T.);
#10886=ORIENTED_EDGE('',*,*,#8076,.F.);
#10887=ORIENTED_EDGE('',*,*,#7880,.F.);
#10888=ORIENTED_EDGE('',*,*,#8081,.T.);
#10889=ORIENTED_EDGE('',*,*,#8082,.T.);
#10890=ORIENTED_EDGE('',*,*,#8079,.F.);
#10891=ORIENTED_EDGE('',*,*,#7879,.F.);
#10892=ORIENTED_EDGE('',*,*,#8078,.T.);
#10893=ORIENTED_EDGE('',*,*,#8083,.T.);
#10894=ORIENTED_EDGE('',*,*,#8081,.F.);
#10895=ORIENTED_EDGE('',*,*,#8083,.F.);
#10896=ORIENTED_EDGE('',*,*,#8077,.F.);
#10897=ORIENTED_EDGE('',*,*,#8080,.F.);
#10898=ORIENTED_EDGE('',*,*,#8082,.F.);
#10899=ORIENTED_EDGE('',*,*,#7874,.F.);
#10900=ORIENTED_EDGE('',*,*,#8084,.T.);
#10901=ORIENTED_EDGE('',*,*,#8085,.T.);
#10902=ORIENTED_EDGE('',*,*,#8086,.F.);
#10903=ORIENTED_EDGE('',*,*,#7877,.F.);
#10904=ORIENTED_EDGE('',*,*,#8087,.T.);
#10905=ORIENTED_EDGE('',*,*,#8088,.T.);
#10906=ORIENTED_EDGE('',*,*,#8084,.F.);
#10907=ORIENTED_EDGE('',*,*,#7876,.F.);
#10908=ORIENTED_EDGE('',*,*,#8089,.T.);
#10909=ORIENTED_EDGE('',*,*,#8090,.T.);
#10910=ORIENTED_EDGE('',*,*,#8087,.F.);
#10911=ORIENTED_EDGE('',*,*,#7875,.F.);
#10912=ORIENTED_EDGE('',*,*,#8086,.T.);
#10913=ORIENTED_EDGE('',*,*,#8091,.T.);
#10914=ORIENTED_EDGE('',*,*,#8089,.F.);
#10915=ORIENTED_EDGE('',*,*,#8091,.F.);
#10916=ORIENTED_EDGE('',*,*,#8085,.F.);
#10917=ORIENTED_EDGE('',*,*,#8088,.F.);
#10918=ORIENTED_EDGE('',*,*,#8090,.F.);
#10919=ORIENTED_EDGE('',*,*,#7870,.F.);
#10920=ORIENTED_EDGE('',*,*,#8092,.T.);
#10921=ORIENTED_EDGE('',*,*,#8093,.T.);
#10922=ORIENTED_EDGE('',*,*,#8094,.F.);
#10923=ORIENTED_EDGE('',*,*,#7873,.F.);
#10924=ORIENTED_EDGE('',*,*,#8095,.T.);
#10925=ORIENTED_EDGE('',*,*,#8096,.T.);
#10926=ORIENTED_EDGE('',*,*,#8092,.F.);
#10927=ORIENTED_EDGE('',*,*,#7872,.F.);
#10928=ORIENTED_EDGE('',*,*,#8097,.T.);
#10929=ORIENTED_EDGE('',*,*,#8098,.T.);
#10930=ORIENTED_EDGE('',*,*,#8095,.F.);
#10931=ORIENTED_EDGE('',*,*,#7871,.F.);
#10932=ORIENTED_EDGE('',*,*,#8094,.T.);
#10933=ORIENTED_EDGE('',*,*,#8099,.T.);
#10934=ORIENTED_EDGE('',*,*,#8097,.F.);
#10935=ORIENTED_EDGE('',*,*,#8099,.F.);
#10936=ORIENTED_EDGE('',*,*,#8093,.F.);
#10937=ORIENTED_EDGE('',*,*,#8096,.F.);
#10938=ORIENTED_EDGE('',*,*,#8098,.F.);
#10939=ORIENTED_EDGE('',*,*,#7642,.F.);
#10940=ORIENTED_EDGE('',*,*,#8100,.T.);
#10941=ORIENTED_EDGE('',*,*,#8101,.T.);
#10942=ORIENTED_EDGE('',*,*,#8100,.F.);
#10943=ORIENTED_EDGE('',*,*,#8102,.T.);
#10944=ORIENTED_EDGE('',*,*,#8101,.F.);
#10945=ORIENTED_EDGE('',*,*,#8102,.F.);
#10946=ORIENTED_EDGE('',*,*,#8103,.T.);
#10947=ORIENTED_EDGE('',*,*,#8104,.T.);
#10948=ORIENTED_EDGE('',*,*,#8103,.F.);
#10949=ORIENTED_EDGE('',*,*,#8104,.F.);
#10950=ORIENTED_EDGE('',*,*,#8105,.T.);
#10951=ORIENTED_EDGE('',*,*,#8105,.F.);
#10952=ORIENTED_EDGE('',*,*,#8106,.T.);
#10953=ORIENTED_EDGE('',*,*,#8107,.T.);
#10954=ORIENTED_EDGE('',*,*,#8106,.F.);
#10955=ORIENTED_EDGE('',*,*,#8107,.F.);
#10956=ORIENTED_EDGE('',*,*,#8108,.T.);
#10957=ORIENTED_EDGE('',*,*,#8108,.F.);
#10958=ORIENTED_EDGE('',*,*,#8109,.T.);
#10959=ORIENTED_EDGE('',*,*,#8110,.F.);
#10960=ORIENTED_EDGE('',*,*,#8111,.F.);
#10961=ORIENTED_EDGE('',*,*,#8112,.T.);
#10962=ORIENTED_EDGE('',*,*,#8113,.T.);
#10963=ORIENTED_EDGE('',*,*,#8112,.F.);
#10964=ORIENTED_EDGE('',*,*,#8114,.F.);
#10965=ORIENTED_EDGE('',*,*,#8109,.F.);
#10966=ORIENTED_EDGE('',*,*,#7839,.T.);
#10967=ORIENTED_EDGE('',*,*,#7840,.T.);
#10968=ORIENTED_EDGE('',*,*,#8115,.T.);
#10969=ORIENTED_EDGE('',*,*,#8113,.F.);
#10970=ORIENTED_EDGE('',*,*,#8115,.F.);
#10971=ORIENTED_EDGE('',*,*,#8116,.T.);
#10972=ORIENTED_EDGE('',*,*,#8117,.T.);
#10973=ORIENTED_EDGE('',*,*,#8116,.F.);
#10974=ORIENTED_EDGE('',*,*,#8118,.T.);
#10975=ORIENTED_EDGE('',*,*,#8117,.F.);
#10976=ORIENTED_EDGE('',*,*,#8118,.F.);
#10977=ORIENTED_EDGE('',*,*,#8119,.T.);
#10978=ORIENTED_EDGE('',*,*,#8120,.T.);
#10979=ORIENTED_EDGE('',*,*,#8119,.F.);
#10980=ORIENTED_EDGE('',*,*,#8120,.F.);
#10981=ORIENTED_EDGE('',*,*,#8121,.T.);
#10982=ORIENTED_EDGE('',*,*,#8121,.F.);
#10983=ORIENTED_EDGE('',*,*,#8122,.T.);
#10984=ORIENTED_EDGE('',*,*,#7745,.F.);
#10985=ORIENTED_EDGE('',*,*,#8122,.F.);
#10986=ORIENTED_EDGE('',*,*,#8018,.F.);
#10987=ORIENTED_EDGE('',*,*,#8123,.T.);
#10988=ORIENTED_EDGE('',*,*,#8124,.T.);
#10989=ORIENTED_EDGE('',*,*,#8123,.F.);
#10990=ORIENTED_EDGE('',*,*,#8110,.T.);
#10991=ORIENTED_EDGE('',*,*,#8114,.T.);
#10992=ORIENTED_EDGE('',*,*,#8111,.T.);
#10993=ORIENTED_EDGE('',*,*,#8124,.F.);
#10994=ORIENTED_EDGE('',*,*,#8125,.T.);
#10995=ORIENTED_EDGE('',*,*,#8125,.F.);
#10996=ORIENTED_EDGE('',*,*,#8126,.T.);
#10997=ORIENTED_EDGE('',*,*,#8127,.T.);
#10998=ORIENTED_EDGE('',*,*,#8126,.F.);
#10999=ORIENTED_EDGE('',*,*,#8127,.F.);
#11000=ORIENTED_EDGE('',*,*,#8128,.T.);
#11001=ORIENTED_EDGE('',*,*,#8128,.F.);
#11002=ORIENTED_EDGE('',*,*,#8129,.T.);
#11003=ORIENTED_EDGE('',*,*,#8130,.T.);
#11004=ORIENTED_EDGE('',*,*,#8129,.F.);
#11005=ORIENTED_EDGE('',*,*,#8130,.F.);
#11006=ORIENTED_EDGE('',*,*,#8131,.T.);
#11007=ORIENTED_EDGE('',*,*,#7834,.F.);
#11008=ORIENTED_EDGE('',*,*,#8131,.F.);
#11009=ORIENTED_EDGE('',*,*,#7806,.F.);
#11010=ORIENTED_EDGE('',*,*,#8035,.F.);
#11011=ORIENTED_EDGE('',*,*,#8045,.F.);
#11012=ORIENTED_EDGE('',*,*,#8036,.T.);
#11013=ORIENTED_EDGE('',*,*,#8038,.T.);
#11014=ORIENTED_EDGE('',*,*,#7634,.T.);
#11015=ORIENTED_EDGE('',*,*,#8017,.T.);
#11016=ORIENTED_EDGE('',*,*,#8050,.T.);
#11017=ORIENTED_EDGE('',*,*,#8044,.T.);
#11018=ORIENTED_EDGE('',*,*,#8051,.T.);
#11019=ORIENTED_EDGE('',*,*,#8011,.T.);
#11020=ORIENTED_EDGE('',*,*,#7742,.T.);
#14459=PLANE('',#15832);
#14460=PLANE('',#15833);
#14461=PLANE('',#15834);
#14462=PLANE('',#15835);
#14463=PLANE('',#15836);
#14464=PLANE('',#15837);
#14465=PLANE('',#15838);
#14466=PLANE('',#15839);
#14467=PLANE('',#15840);
#14468=PLANE('',#15841);
#14469=PLANE('',#15842);
#14470=PLANE('',#15843);
#14471=PLANE('',#15844);
#14472=PLANE('',#15845);
#14473=PLANE('',#15846);
#14474=PLANE('',#15847);
#14475=PLANE('',#15848);
#14476=PLANE('',#15849);
#14477=PLANE('',#15850);
#14478=PLANE('',#15851);
#14479=PLANE('',#15852);
#14480=PLANE('',#15853);
#14481=PLANE('',#15854);
#14482=PLANE('',#15855);
#14483=PLANE('',#15856);
#14484=PLANE('',#15857);
#14485=PLANE('',#15858);
#14486=PLANE('',#15859);
#14487=PLANE('',#15860);
#14488=PLANE('',#15861);
#14489=PLANE('',#15862);
#14490=PLANE('',#15863);
#14491=PLANE('',#15864);
#14492=PLANE('',#15866);
#14493=PLANE('',#15867);
#14494=PLANE('',#15868);
#14495=PLANE('',#15869);
#14496=PLANE('',#15870);
#14497=PLANE('',#15871);
#14498=PLANE('',#15872);
#14499=PLANE('',#15873);
#14500=PLANE('',#15874);
#14501=PLANE('',#15875);
#14502=PLANE('',#15876);
#14503=PLANE('',#15877);
#14504=PLANE('',#15878);
#14505=PLANE('',#15879);
#14506=PLANE('',#15880);
#14507=PLANE('',#15881);
#14508=PLANE('',#15882);
#14509=PLANE('',#15883);
#14510=PLANE('',#15884);
#14511=PLANE('',#15885);
#14512=PLANE('',#15886);
#14513=PLANE('',#15887);
#14514=PLANE('',#15888);
#14515=PLANE('',#15889);
#14516=PLANE('',#15890);
#14517=PLANE('',#15891);
#14518=PLANE('',#15892);
#14519=PLANE('',#15893);
#14520=PLANE('',#15894);
#14521=PLANE('',#15895);
#14522=PLANE('',#15896);
#14523=PLANE('',#15897);
#14524=PLANE('',#15898);
#14525=PLANE('',#15912);
#14526=PLANE('',#15913);
#14527=PLANE('',#15914);
#14528=PLANE('',#15918);
#14529=PLANE('',#15919);
#14530=PLANE('',#15920);
#14531=PLANE('',#15921);
#14532=PLANE('',#15922);
#14533=PLANE('',#15926);
#14534=PLANE('',#15942);
#14535=PLANE('',#15954);
#14536=PLANE('',#15977);
#14537=PLANE('',#15994);
#14538=PLANE('',#16104);
#14539=PLANE('',#16105);
#14540=PLANE('',#16106);
#14541=PLANE('',#16107);
#14542=PLANE('',#16108);
#14543=PLANE('',#16109);
#14544=PLANE('',#16113);
#14545=PLANE('',#16114);
#14546=PLANE('',#16115);
#14547=PLANE('',#16116);
#14548=PLANE('',#16117);
#14549=PLANE('',#16118);
#14550=PLANE('',#16119);
#14551=PLANE('',#16125);
#14552=PLANE('',#16129);
#14553=PLANE('',#16130);
#14554=PLANE('',#16131);
#14555=PLANE('',#16132);
#14556=PLANE('',#16133);
#14557=PLANE('',#16134);
#14558=PLANE('',#16135);
#14559=PLANE('',#16136);
#14560=PLANE('',#16137);
#14561=PLANE('',#16138);
#14562=PLANE('',#16139);
#14563=PLANE('',#16140);
#14564=PLANE('',#16141);
#14565=PLANE('',#16142);
#14566=PLANE('',#16143);
#14567=PLANE('',#16144);
#14568=PLANE('',#16145);
#14569=PLANE('',#16146);
#14570=PLANE('',#16147);
#14571=PLANE('',#16148);
#14572=PLANE('',#16149);
#14573=PLANE('',#16150);
#14574=PLANE('',#16151);
#14575=PLANE('',#16152);
#14576=PLANE('',#16153);
#14577=PLANE('',#16154);
#14578=PLANE('',#16155);
#14579=PLANE('',#16156);
#14580=PLANE('',#16157);
#14581=PLANE('',#16158);
#14582=PLANE('',#16159);
#14583=PLANE('',#16160);
#14584=PLANE('',#16161);
#14585=PLANE('',#16162);
#14586=PLANE('',#16163);
#14587=PLANE('',#16166);
#14588=PLANE('',#16170);
#14589=PLANE('',#16174);
#14590=PLANE('',#16178);
#14591=PLANE('',#16182);
#14592=PLANE('',#16186);
#14593=PLANE('',#16191);
#14594=PLANE('',#16195);
#14741=ADVANCED_FACE('',(#2385),#14459,.F.);
#14742=ADVANCED_FACE('',(#2386),#14460,.F.);
#14743=ADVANCED_FACE('',(#2387),#14461,.F.);
#14744=ADVANCED_FACE('',(#2388),#14462,.F.);
#14745=ADVANCED_FACE('',(#2389),#14463,.F.);
#14746=ADVANCED_FACE('',(#2390),#14464,.F.);
#14747=ADVANCED_FACE('',(#2391),#14465,.F.);
#14748=ADVANCED_FACE('',(#2392),#14466,.F.);
#14749=ADVANCED_FACE('',(#2393),#14467,.F.);
#14750=ADVANCED_FACE('',(#2394),#14468,.F.);
#14751=ADVANCED_FACE('',(#2395),#14469,.F.);
#14752=ADVANCED_FACE('',(#2396),#14470,.F.);
#14753=ADVANCED_FACE('',(#2397),#14471,.F.);
#14754=ADVANCED_FACE('',(#2398),#14472,.F.);
#14755=ADVANCED_FACE('',(#2399),#14473,.F.);
#14756=ADVANCED_FACE('',(#2400),#14474,.F.);
#14757=ADVANCED_FACE('',(#2401),#14475,.F.);
#14758=ADVANCED_FACE('',(#2402),#14476,.F.);
#14759=ADVANCED_FACE('',(#2403),#14477,.F.);
#14760=ADVANCED_FACE('',(#2404),#14478,.F.);
#14761=ADVANCED_FACE('',(#2405),#14479,.F.);
#14762=ADVANCED_FACE('',(#2406),#14480,.F.);
#14763=ADVANCED_FACE('',(#2407),#14481,.F.);
#14764=ADVANCED_FACE('',(#2408),#14482,.F.);
#14765=ADVANCED_FACE('',(#2409),#14483,.F.);
#14766=ADVANCED_FACE('',(#2410),#14484,.F.);
#14767=ADVANCED_FACE('',(#2411),#14485,.F.);
#14768=ADVANCED_FACE('',(#2412),#14486,.F.);
#14769=ADVANCED_FACE('',(#2413),#14487,.F.);
#14770=ADVANCED_FACE('',(#2414),#14488,.F.);
#14771=ADVANCED_FACE('',(#2415),#14489,.F.);
#14772=ADVANCED_FACE('',(#2416),#14490,.F.);
#14773=ADVANCED_FACE('',(#2417,#1602,#1603,#1604,#1605,#1606),#14491,.T.);
#14774=ADVANCED_FACE('',(#2418),#14492,.F.);
#14775=ADVANCED_FACE('',(#2419),#14493,.F.);
#14776=ADVANCED_FACE('',(#2420),#14494,.F.);
#14777=ADVANCED_FACE('',(#2421),#14495,.F.);
#14778=ADVANCED_FACE('',(#2422),#14496,.F.);
#14779=ADVANCED_FACE('',(#2423),#14497,.F.);
#14780=ADVANCED_FACE('',(#2424),#14498,.F.);
#14781=ADVANCED_FACE('',(#2425),#14499,.F.);
#14782=ADVANCED_FACE('',(#2426),#14500,.F.);
#14783=ADVANCED_FACE('',(#2427),#14501,.F.);
#14784=ADVANCED_FACE('',(#2428),#14502,.F.);
#14785=ADVANCED_FACE('',(#2429),#14503,.F.);
#14786=ADVANCED_FACE('',(#2430),#14504,.F.);
#14787=ADVANCED_FACE('',(#2431),#14505,.F.);
#14788=ADVANCED_FACE('',(#2432),#14506,.F.);
#14789=ADVANCED_FACE('',(#2433),#14507,.F.);
#14790=ADVANCED_FACE('',(#2434),#14508,.F.);
#14791=ADVANCED_FACE('',(#2435),#14509,.F.);
#14792=ADVANCED_FACE('',(#2436),#14510,.F.);
#14793=ADVANCED_FACE('',(#2437),#14511,.F.);
#14794=ADVANCED_FACE('',(#2438),#14512,.F.);
#14795=ADVANCED_FACE('',(#2439),#14513,.F.);
#14796=ADVANCED_FACE('',(#2440),#14514,.F.);
#14797=ADVANCED_FACE('',(#2441),#14515,.F.);
#14798=ADVANCED_FACE('',(#2442),#14516,.F.);
#14799=ADVANCED_FACE('',(#2443),#14517,.F.);
#14800=ADVANCED_FACE('',(#2444),#14518,.F.);
#14801=ADVANCED_FACE('',(#2445),#14519,.F.);
#14802=ADVANCED_FACE('',(#2446),#14520,.F.);
#14803=ADVANCED_FACE('',(#2447),#14521,.F.);
#14804=ADVANCED_FACE('',(#2448),#14522,.F.);
#14805=ADVANCED_FACE('',(#2449),#14523,.F.);
#14806=ADVANCED_FACE('',(#2450,#1607,#1608,#1609,#1610,#1611,#1612,#1613),
#14524,.T.);
#14807=ADVANCED_FACE('',(#2451),#1351,.T.);
#14808=ADVANCED_FACE('',(#2452),#1352,.T.);
#14809=ADVANCED_FACE('',(#2453),#14525,.F.);
#14810=ADVANCED_FACE('',(#2454),#14526,.F.);
#14811=ADVANCED_FACE('',(#2455),#14527,.F.);
#14812=ADVANCED_FACE('',(#2456),#1353,.T.);
#14813=ADVANCED_FACE('',(#2457),#14528,.F.);
#14814=ADVANCED_FACE('',(#2458),#14529,.F.);
#14815=ADVANCED_FACE('',(#2459),#14530,.F.);
#14816=ADVANCED_FACE('',(#2460),#14531,.F.);
#14817=ADVANCED_FACE('',(#2461),#14532,.T.);
#14818=ADVANCED_FACE('',(#2462),#14533,.T.);
#14819=ADVANCED_FACE('',(#2463),#1145,.T.);
#14820=ADVANCED_FACE('',(#2464),#1146,.T.);
#14821=ADVANCED_FACE('',(#2465),#14534,.T.);
#14822=ADVANCED_FACE('',(#2466),#1147,.T.);
#14823=ADVANCED_FACE('',(#2467),#1148,.T.);
#14824=ADVANCED_FACE('',(#2468),#1149,.T.);
#14825=ADVANCED_FACE('',(#2469),#14535,.T.);
#14826=ADVANCED_FACE('',(#2470),#1150,.T.);
#14827=ADVANCED_FACE('',(#2471),#1151,.T.);
#14828=ADVANCED_FACE('',(#2472),#1152,.T.);
#14829=ADVANCED_FACE('',(#2473),#1153,.T.);
#14830=ADVANCED_FACE('',(#2474),#1154,.T.);
#14831=ADVANCED_FACE('',(#2475),#1354,.T.);
#14832=ADVANCED_FACE('',(#2476),#1355,.T.);
#14833=ADVANCED_FACE('',(#2477),#1356,.T.);
#14834=ADVANCED_FACE('',(#2478),#1357,.T.);
#14835=ADVANCED_FACE('',(#2479),#1358,.T.);
#14836=ADVANCED_FACE('',(#2480),#1359,.T.);
#14837=ADVANCED_FACE('',(#2481,#1614,#1615,#1616,#1617,#1618),#14536,.T.);
#14838=ADVANCED_FACE('',(#2482),#1360,.F.);
#14839=ADVANCED_FACE('',(#2483),#1155,.F.);
#14840=ADVANCED_FACE('',(#2484),#1156,.F.);
#14841=ADVANCED_FACE('',(#2485),#1361,.F.);
#14842=ADVANCED_FACE('',(#2486),#1157,.F.);
#14843=ADVANCED_FACE('',(#2487,#1619,#1620,#1621,#1622,#1623,#1624,#1625),
#14537,.T.);
#14844=ADVANCED_FACE('',(#2488),#1158,.F.);
#14845=ADVANCED_FACE('',(#2489,#1626),#1362,.F.);
#14846=ADVANCED_FACE('',(#2490),#1159,.F.);
#14847=ADVANCED_FACE('',(#2491),#1363,.T.);
#14848=ADVANCED_FACE('',(#2492),#1160,.F.);
#14849=ADVANCED_FACE('',(#2493),#1364,.F.);
#14850=ADVANCED_FACE('',(#2494),#1161,.F.);
#14851=ADVANCED_FACE('',(#2495),#1365,.T.);
#14852=ADVANCED_FACE('',(#2496),#1162,.F.);
#14853=ADVANCED_FACE('',(#2497),#1366,.F.);
#14854=ADVANCED_FACE('',(#2498),#1163,.F.);
#14855=ADVANCED_FACE('',(#2499),#1164,.F.);
#14856=ADVANCED_FACE('',(#2500),#1367,.F.);
#14857=ADVANCED_FACE('',(#2501),#1165,.F.);
#14858=ADVANCED_FACE('',(#2502),#1166,.F.);
#14859=ADVANCED_FACE('',(#2503),#1368,.F.);
#14860=ADVANCED_FACE('',(#2504),#1167,.F.);
#14861=ADVANCED_FACE('',(#2505),#1168,.F.);
#14862=ADVANCED_FACE('',(#2506),#1369,.F.);
#14863=ADVANCED_FACE('',(#2507),#1169,.F.);
#14864=ADVANCED_FACE('',(#2508),#1170,.F.);
#14865=ADVANCED_FACE('',(#2509),#1370,.F.);
#14866=ADVANCED_FACE('',(#2510),#1171,.F.);
#14867=ADVANCED_FACE('',(#2511),#1172,.F.);
#14868=ADVANCED_FACE('',(#2512),#1371,.F.);
#14869=ADVANCED_FACE('',(#2513),#1173,.F.);
#14870=ADVANCED_FACE('',(#2514),#1174,.F.);
#14871=ADVANCED_FACE('',(#2515),#1372,.F.);
#14872=ADVANCED_FACE('',(#2516),#1175,.F.);
#14873=ADVANCED_FACE('',(#2517),#1176,.F.);
#14874=ADVANCED_FACE('',(#2518),#1373,.F.);
#14875=ADVANCED_FACE('',(#2519),#1177,.F.);
#14876=ADVANCED_FACE('',(#2520),#1178,.F.);
#14877=ADVANCED_FACE('',(#2521),#1374,.F.);
#14878=ADVANCED_FACE('',(#2522),#1179,.F.);
#14879=ADVANCED_FACE('',(#2523),#1180,.F.);
#14880=ADVANCED_FACE('',(#2524),#1375,.F.);
#14881=ADVANCED_FACE('',(#2525),#1181,.F.);
#14882=ADVANCED_FACE('',(#2526),#1182,.F.);
#14883=ADVANCED_FACE('',(#2527),#1376,.F.);
#14884=ADVANCED_FACE('',(#2528),#1183,.F.);
#14885=ADVANCED_FACE('',(#2529),#1184,.F.);
#14886=ADVANCED_FACE('',(#2530,#1627),#1377,.F.);
#14887=ADVANCED_FACE('',(#2531),#1185,.F.);
#14888=ADVANCED_FACE('',(#2532),#1186,.F.);
#14889=ADVANCED_FACE('',(#2533),#1378,.F.);
#14890=ADVANCED_FACE('',(#2534),#1187,.F.);
#14891=ADVANCED_FACE('',(#2535),#1379,.F.);
#14892=ADVANCED_FACE('',(#2536),#1188,.F.);
#14893=ADVANCED_FACE('',(#2537),#1380,.F.);
#14894=ADVANCED_FACE('',(#2538),#1189,.F.);
#14895=ADVANCED_FACE('',(#2539),#1381,.F.);
#14896=ADVANCED_FACE('',(#2540),#1190,.F.);
#14897=ADVANCED_FACE('',(#2541),#1382,.F.);
#14898=ADVANCED_FACE('',(#2542),#1191,.F.);
#14899=ADVANCED_FACE('',(#2543),#14538,.F.);
#14900=ADVANCED_FACE('',(#2544,#1628),#14539,.F.);
#14901=ADVANCED_FACE('',(#2545),#14540,.F.);
#14902=ADVANCED_FACE('',(#2546),#14541,.F.);
#14903=ADVANCED_FACE('',(#2547,#1629),#14542,.F.);
#14904=ADVANCED_FACE('',(#2548,#1630,#1631,#1632,#1633,#1634,#1635),#14543,
 .T.);
#14905=ADVANCED_FACE('',(#2549,#1636),#14544,.F.);
#14906=ADVANCED_FACE('',(#2550),#14545,.T.);
#14907=ADVANCED_FACE('',(#2551),#14546,.F.);
#14908=ADVANCED_FACE('',(#2552),#14547,.F.);
#14909=ADVANCED_FACE('',(#2553),#14548,.F.);
#14910=ADVANCED_FACE('',(#2554,#1637),#14549,.F.);
#14911=ADVANCED_FACE('',(#2555),#14550,.T.);
#14912=ADVANCED_FACE('',(#2556),#1383,.T.);
#14913=ADVANCED_FACE('',(#2557),#1384,.T.);
#14914=ADVANCED_FACE('',(#2558),#1385,.T.);
#14915=ADVANCED_FACE('',(#2559),#14551,.T.);
#14916=ADVANCED_FACE('',(#2560),#14552,.F.);
#14917=ADVANCED_FACE('',(#2561),#14553,.F.);
#14918=ADVANCED_FACE('',(#2562),#14554,.F.);
#14919=ADVANCED_FACE('',(#2563,#1638,#1639),#14555,.T.);
#14920=ADVANCED_FACE('',(#2564,#1640,#1641),#14556,.T.);
#14921=ADVANCED_FACE('',(#2565),#14557,.F.);
#14922=ADVANCED_FACE('',(#2566),#14558,.F.);
#14923=ADVANCED_FACE('',(#2567),#14559,.F.);
#14924=ADVANCED_FACE('',(#2568),#14560,.F.);
#14925=ADVANCED_FACE('',(#2569),#14561,.F.);
#14926=ADVANCED_FACE('',(#2570),#14562,.F.);
#14927=ADVANCED_FACE('',(#2571),#14563,.F.);
#14928=ADVANCED_FACE('',(#2572),#14564,.F.);
#14929=ADVANCED_FACE('',(#2573),#14565,.F.);
#14930=ADVANCED_FACE('',(#2574),#14566,.F.);
#14931=ADVANCED_FACE('',(#2575),#14567,.F.);
#14932=ADVANCED_FACE('',(#2576),#14568,.F.);
#14933=ADVANCED_FACE('',(#2577),#14569,.F.);
#14934=ADVANCED_FACE('',(#2578),#14570,.F.);
#14935=ADVANCED_FACE('',(#2579),#14571,.F.);
#14936=ADVANCED_FACE('',(#2580),#14572,.F.);
#14937=ADVANCED_FACE('',(#2581),#14573,.F.);
#14938=ADVANCED_FACE('',(#2582),#14574,.F.);
#14939=ADVANCED_FACE('',(#2583),#14575,.F.);
#14940=ADVANCED_FACE('',(#2584),#14576,.F.);
#14941=ADVANCED_FACE('',(#2585),#14577,.F.);
#14942=ADVANCED_FACE('',(#2586),#14578,.F.);
#14943=ADVANCED_FACE('',(#2587),#14579,.F.);
#14944=ADVANCED_FACE('',(#2588),#14580,.F.);
#14945=ADVANCED_FACE('',(#2589),#14581,.F.);
#14946=ADVANCED_FACE('',(#2590),#14582,.F.);
#14947=ADVANCED_FACE('',(#2591),#14583,.F.);
#14948=ADVANCED_FACE('',(#2592),#14584,.F.);
#14949=ADVANCED_FACE('',(#2593),#14585,.F.);
#14950=ADVANCED_FACE('',(#2594),#14586,.F.);
#14951=ADVANCED_FACE('',(#2595),#1386,.F.);
#14952=ADVANCED_FACE('',(#2596,#1642),#14587,.F.);
#14953=ADVANCED_FACE('',(#2597),#1387,.F.);
#14954=ADVANCED_FACE('',(#2598,#1643),#14588,.F.);
#14955=ADVANCED_FACE('',(#2599),#1388,.F.);
#14956=ADVANCED_FACE('',(#2600,#1644),#14589,.F.);
#14957=ADVANCED_FACE('',(#2601,#1645),#1389,.F.);
#14958=ADVANCED_FACE('',(#2602,#1646),#14590,.F.);
#14959=ADVANCED_FACE('',(#2603),#1390,.F.);
#14960=ADVANCED_FACE('',(#2604,#1647),#14591,.F.);
#14961=ADVANCED_FACE('',(#2605),#1391,.F.);
#14962=ADVANCED_FACE('',(#2606,#1648),#14592,.F.);
#14963=ADVANCED_FACE('',(#2607),#1392,.F.);
#14964=ADVANCED_FACE('',(#2608,#1649),#1393,.F.);
#14965=ADVANCED_FACE('',(#2609,#1650),#14593,.F.);
#14966=ADVANCED_FACE('',(#2610),#1394,.F.);
#14967=ADVANCED_FACE('',(#2611,#1651),#14594,.F.);
#14968=ADVANCED_FACE('',(#2612),#1395,.F.);
#14969=ADVANCED_FACE('',(#2613),#1192,.F.);
#14970=ADVANCED_FACE('',(#2614),#1396,.T.);
#14971=ADVANCED_FACE('',(#2615),#1397,.T.);
#14972=ADVANCED_FACE('',(#2616),#1398,.T.);
#15613=CLOSED_SHELL('',(#14741,#14742,#14743,#14744,#14745,#14746,#14747,
#14748,#14749,#14750,#14751,#14752,#14753,#14754,#14755,#14756,#14757,#14758,
#14759,#14760,#14761,#14762,#14763,#14764,#14765,#14766,#14767,#14768,#14769,
#14770,#14771,#14772,#14773,#14774,#14775,#14776,#14777,#14778,#14779,#14780,
#14781,#14782,#14783,#14784,#14785,#14786,#14787,#14788,#14789,#14790,#14791,
#14792,#14793,#14794,#14795,#14796,#14797,#14798,#14799,#14800,#14801,#14802,
#14803,#14804,#14805,#14806,#14807,#14808,#14809,#14810,#14811,#14812,#14813,
#14814,#14815,#14816,#14817,#14818,#14819,#14820,#14821,#14822,#14823,#14824,
#14825,#14826,#14827,#14828,#14829,#14830,#14831,#14832,#14833,#14834,#14835,
#14836,#14837,#14838,#14839,#14840,#14841,#14842,#14843,#14844,#14845,#14846,
#14847,#14848,#14849,#14850,#14851,#14852,#14853,#14854,#14855,#14856,#14857,
#14858,#14859,#14860,#14861,#14862,#14863,#14864,#14865,#14866,#14867,#14868,
#14869,#14870,#14871,#14872,#14873,#14874,#14875,#14876,#14877,#14878,#14879,
#14880,#14881,#14882,#14883,#14884,#14885,#14886,#14887,#14888,#14889,#14890,
#14891,#14892,#14893,#14894,#14895,#14896,#14897,#14898,#14899,#14900,#14901,
#14902,#14903,#14904,#14905,#14906,#14907,#14908,#14909,#14910,#14911,#14912,
#14913,#14914,#14915,#14916,#14917,#14918,#14919,#14920,#14921,#14922,#14923,
#14924,#14925,#14926,#14927,#14928,#14929,#14930,#14931,#14932,#14933,#14934,
#14935,#14936,#14937,#14938,#14939,#14940,#14941,#14942,#14943,#14944,#14945,
#14946,#14947,#14948,#14949,#14950,#14951,#14952,#14953,#14954,#14955,#14956,
#14957,#14958,#14959,#14960,#14961,#14962,#14963,#14964,#14965,#14966,#14967,
#14968,#14969,#14970,#14971,#14972));
#15831=AXIS2_PLACEMENT_3D('',#21059,#17288,#17289);
#15832=AXIS2_PLACEMENT_3D('',#21060,#17290,#17291);
#15833=AXIS2_PLACEMENT_3D('',#21069,#17296,#17297);
#15834=AXIS2_PLACEMENT_3D('',#21075,#17301,#17302);
#15835=AXIS2_PLACEMENT_3D('',#21081,#17306,#17307);
#15836=AXIS2_PLACEMENT_3D('',#21084,#17310,#17311);
#15837=AXIS2_PLACEMENT_3D('',#21085,#17312,#17313);
#15838=AXIS2_PLACEMENT_3D('',#21094,#17318,#17319);
#15839=AXIS2_PLACEMENT_3D('',#21104,#17325,#17326);
#15840=AXIS2_PLACEMENT_3D('',#21108,#17329,#17330);
#15841=AXIS2_PLACEMENT_3D('',#21112,#17333,#17334);
#15842=AXIS2_PLACEMENT_3D('',#21116,#17337,#17338);
#15843=AXIS2_PLACEMENT_3D('',#21125,#17343,#17344);
#15844=AXIS2_PLACEMENT_3D('',#21131,#17348,#17349);
#15845=AXIS2_PLACEMENT_3D('',#21137,#17353,#17354);
#15846=AXIS2_PLACEMENT_3D('',#21140,#17357,#17358);
#15847=AXIS2_PLACEMENT_3D('',#21141,#17359,#17360);
#15848=AXIS2_PLACEMENT_3D('',#21150,#17365,#17366);
#15849=AXIS2_PLACEMENT_3D('',#21156,#17370,#17371);
#15850=AXIS2_PLACEMENT_3D('',#21162,#17375,#17376);
#15851=AXIS2_PLACEMENT_3D('',#21165,#17379,#17380);
#15852=AXIS2_PLACEMENT_3D('',#21166,#17381,#17382);
#15853=AXIS2_PLACEMENT_3D('',#21175,#17387,#17388);
#15854=AXIS2_PLACEMENT_3D('',#21181,#17392,#17393);
#15855=AXIS2_PLACEMENT_3D('',#21187,#17397,#17398);
#15856=AXIS2_PLACEMENT_3D('',#21190,#17401,#17402);
#15857=AXIS2_PLACEMENT_3D('',#21191,#17403,#17404);
#15858=AXIS2_PLACEMENT_3D('',#21200,#17409,#17410);
#15859=AXIS2_PLACEMENT_3D('',#21209,#17415,#17416);
#15860=AXIS2_PLACEMENT_3D('',#21215,#17420,#17421);
#15861=AXIS2_PLACEMENT_3D('',#21218,#17424,#17425);
#15862=AXIS2_PLACEMENT_3D('',#21222,#17428,#17429);
#15863=AXIS2_PLACEMENT_3D('',#21230,#17434,#17435);
#15864=AXIS2_PLACEMENT_3D('',#21236,#17439,#17440);
#15865=AXIS2_PLACEMENT_3D('',#21256,#17451,#17452);
#15866=AXIS2_PLACEMENT_3D('',#21257,#17453,#17454);
#15867=AXIS2_PLACEMENT_3D('',#21266,#17459,#17460);
#15868=AXIS2_PLACEMENT_3D('',#21272,#17464,#17465);
#15869=AXIS2_PLACEMENT_3D('',#21278,#17469,#17470);
#15870=AXIS2_PLACEMENT_3D('',#21281,#17473,#17474);
#15871=AXIS2_PLACEMENT_3D('',#21282,#17475,#17476);
#15872=AXIS2_PLACEMENT_3D('',#21291,#17481,#17482);
#15873=AXIS2_PLACEMENT_3D('',#21300,#17487,#17488);
#15874=AXIS2_PLACEMENT_3D('',#21303,#17491,#17492);
#15875=AXIS2_PLACEMENT_3D('',#21309,#17496,#17497);
#15876=AXIS2_PLACEMENT_3D('',#21313,#17500,#17501);
#15877=AXIS2_PLACEMENT_3D('',#21322,#17506,#17507);
#15878=AXIS2_PLACEMENT_3D('',#21328,#17511,#17512);
#15879=AXIS2_PLACEMENT_3D('',#21334,#17516,#17517);
#15880=AXIS2_PLACEMENT_3D('',#21337,#17520,#17521);
#15881=AXIS2_PLACEMENT_3D('',#21338,#17522,#17523);
#15882=AXIS2_PLACEMENT_3D('',#21347,#17528,#17529);
#15883=AXIS2_PLACEMENT_3D('',#21353,#17533,#17534);
#15884=AXIS2_PLACEMENT_3D('',#21359,#17538,#17539);
#15885=AXIS2_PLACEMENT_3D('',#21362,#17542,#17543);
#15886=AXIS2_PLACEMENT_3D('',#21363,#17544,#17545);
#15887=AXIS2_PLACEMENT_3D('',#21372,#17550,#17551);
#15888=AXIS2_PLACEMENT_3D('',#21378,#17555,#17556);
#15889=AXIS2_PLACEMENT_3D('',#21384,#17560,#17561);
#15890=AXIS2_PLACEMENT_3D('',#21387,#17564,#17565);
#15891=AXIS2_PLACEMENT_3D('',#21388,#17566,#17567);
#15892=AXIS2_PLACEMENT_3D('',#21397,#17572,#17573);
#15893=AXIS2_PLACEMENT_3D('',#21403,#17577,#17578);
#15894=AXIS2_PLACEMENT_3D('',#21412,#17583,#17584);
#15895=AXIS2_PLACEMENT_3D('',#21415,#17587,#17588);
#15896=AXIS2_PLACEMENT_3D('',#21419,#17591,#17592);
#15897=AXIS2_PLACEMENT_3D('',#21427,#17597,#17598);
#15898=AXIS2_PLACEMENT_3D('',#21435,#17603,#17604);
#15899=AXIS2_PLACEMENT_3D('',#21443,#17608,#17609);
#15900=AXIS2_PLACEMENT_3D('',#21445,#17610,#17611);
#15901=AXIS2_PLACEMENT_3D('',#21449,#17613,#17614);
#15902=AXIS2_PLACEMENT_3D('',#21451,#17615,#17616);
#15903=AXIS2_PLACEMENT_3D('',#21467,#17625,#17626);
#15904=AXIS2_PLACEMENT_3D('',#21469,#17627,#17628);
#15905=AXIS2_PLACEMENT_3D('',#21471,#17629,#17630);
#15906=AXIS2_PLACEMENT_3D('',#21472,#17631,#17632);
#15907=AXIS2_PLACEMENT_3D('',#21475,#17633,#17634);
#15908=AXIS2_PLACEMENT_3D('',#21479,#17636,#17637);
#15909=AXIS2_PLACEMENT_3D('',#21481,#17639,#17640);
#15910=AXIS2_PLACEMENT_3D('',#21483,#17641,#17642);
#15911=AXIS2_PLACEMENT_3D('',#21486,#17644,#17645);
#15912=AXIS2_PLACEMENT_3D('',#21487,#17646,#17647);
#15913=AXIS2_PLACEMENT_3D('',#21493,#17651,#17652);
#15914=AXIS2_PLACEMENT_3D('',#21499,#17656,#17657);
#15915=AXIS2_PLACEMENT_3D('',#21505,#17661,#17662);
#15916=AXIS2_PLACEMENT_3D('',#21506,#17663,#17664);
#15917=AXIS2_PLACEMENT_3D('',#21507,#17665,#17666);
#15918=AXIS2_PLACEMENT_3D('',#21508,#17667,#17668);
#15919=AXIS2_PLACEMENT_3D('',#21509,#17669,#17670);
#15920=AXIS2_PLACEMENT_3D('',#21518,#17675,#17676);
#15921=AXIS2_PLACEMENT_3D('',#21524,#17680,#17681);
#15922=AXIS2_PLACEMENT_3D('',#21530,#17685,#17686);
#15923=AXIS2_PLACEMENT_3D('',#21532,#17687,#17688);
#15924=AXIS2_PLACEMENT_3D('',#21534,#17689,#17690);
#15925=AXIS2_PLACEMENT_3D('',#21535,#17691,#17692);
#15926=AXIS2_PLACEMENT_3D('',#21536,#17693,#17694);
#15927=AXIS2_PLACEMENT_3D('',#21538,#17695,#17696);
#15928=AXIS2_PLACEMENT_3D('',#21540,#17697,#17698);
#15929=AXIS2_PLACEMENT_3D('',#21542,#17699,#17700);
#15930=AXIS2_PLACEMENT_3D('',#21545,#17702,#17703);
#15931=AXIS2_PLACEMENT_3D('',#21548,#17705,#17706);
#15932=AXIS2_PLACEMENT_3D('',#21554,#17709,#17710);
#15933=AXIS2_PLACEMENT_3D('',#21556,#17711,#17712);
#15934=AXIS2_PLACEMENT_3D('',#21557,#17713,#17714);
#15935=AXIS2_PLACEMENT_3D('',#21558,#17715,#17716);
#15936=AXIS2_PLACEMENT_3D('',#21561,#17717,#17718);
#15937=AXIS2_PLACEMENT_3D('',#21568,#17719,#17720);
#15938=AXIS2_PLACEMENT_3D('',#21573,#17721,#17722);
#15939=AXIS2_PLACEMENT_3D('',#21575,#17723,#17724);
#15940=AXIS2_PLACEMENT_3D('',#21577,#17725,#17726);
#15941=AXIS2_PLACEMENT_3D('',#21578,#17727,#17728);
#15942=AXIS2_PLACEMENT_3D('',#21579,#17729,#17730);
#15943=AXIS2_PLACEMENT_3D('',#21583,#17732,#17733);
#15944=AXIS2_PLACEMENT_3D('',#21585,#17735,#17736);
#15945=AXIS2_PLACEMENT_3D('',#21587,#17737,#17738);
#15946=AXIS2_PLACEMENT_3D('',#21593,#17739,#17740);
#15947=AXIS2_PLACEMENT_3D('',#21594,#17741,#17742);
#15948=AXIS2_PLACEMENT_3D('',#21596,#17743,#17744);
#15949=AXIS2_PLACEMENT_3D('',#21602,#17745,#17746);
#15950=AXIS2_PLACEMENT_3D('',#21603,#17747,#17748);
#15951=AXIS2_PLACEMENT_3D('',#21605,#17749,#17750);
#15952=AXIS2_PLACEMENT_3D('',#21607,#17751,#17752);
#15953=AXIS2_PLACEMENT_3D('',#21608,#17753,#17754);
#15954=AXIS2_PLACEMENT_3D('',#21609,#17755,#17756);
#15955=AXIS2_PLACEMENT_3D('',#21613,#17758,#17759);
#15956=AXIS2_PLACEMENT_3D('',#21615,#17761,#17762);
#15957=AXIS2_PLACEMENT_3D('',#21617,#17763,#17764);
#15958=AXIS2_PLACEMENT_3D('',#21619,#17765,#17766);
#15959=AXIS2_PLACEMENT_3D('',#21624,#17767,#17768);
#15960=AXIS2_PLACEMENT_3D('',#21626,#17769,#17770);
#15961=AXIS2_PLACEMENT_3D('',#21628,#17771,#17772);
#15962=AXIS2_PLACEMENT_3D('',#21633,#17773,#17774);
#15963=AXIS2_PLACEMENT_3D('',#21635,#17775,#17776);
#15964=AXIS2_PLACEMENT_3D('',#21637,#17777,#17778);
#15965=AXIS2_PLACEMENT_3D('',#21642,#17779,#17780);
#15966=AXIS2_PLACEMENT_3D('',#21644,#17781,#17782);
#15967=AXIS2_PLACEMENT_3D('',#21646,#17783,#17784);
#15968=AXIS2_PLACEMENT_3D('',#21651,#17785,#17786);
#15969=AXIS2_PLACEMENT_3D('',#21652,#17787,#17788);
#15970=AXIS2_PLACEMENT_3D('',#21653,#17789,#17790);
#15971=AXIS2_PLACEMENT_3D('',#21654,#17791,#17792);
#15972=AXIS2_PLACEMENT_3D('',#21657,#17795,#17796);
#15973=AXIS2_PLACEMENT_3D('',#21659,#17798,#17799);
#15974=AXIS2_PLACEMENT_3D('',#21661,#17801,#17802);
#15975=AXIS2_PLACEMENT_3D('',#21663,#17804,#17805);
#15976=AXIS2_PLACEMENT_3D('',#21665,#17807,#17808);
#15977=AXIS2_PLACEMENT_3D('',#21667,#17810,#17811);
#15978=AXIS2_PLACEMENT_3D('',#21669,#17812,#17813);
#15979=AXIS2_PLACEMENT_3D('',#21671,#17814,#17815);
#15980=AXIS2_PLACEMENT_3D('',#21673,#17816,#17817);
#15981=AXIS2_PLACEMENT_3D('',#21675,#17818,#17819);
#15982=AXIS2_PLACEMENT_3D('',#21677,#17820,#17821);
#15983=AXIS2_PLACEMENT_3D('',#21678,#17822,#17823);
#15984=AXIS2_PLACEMENT_3D('',#21719,#17825,#17826);
#15985=AXIS2_PLACEMENT_3D('',#21720,#17827,#17828);
#15986=AXIS2_PLACEMENT_3D('',#21723,#17830,#17831);
#15987=AXIS2_PLACEMENT_3D('',#21724,#17832,#17833);
#15988=AXIS2_PLACEMENT_3D('',#21728,#17835,#17836);
#15989=AXIS2_PLACEMENT_3D('',#21729,#17837,#17838);
#15990=AXIS2_PLACEMENT_3D('',#21764,#17841,#17842);
#15991=AXIS2_PLACEMENT_3D('',#21792,#17843,#17844);
#15992=AXIS2_PLACEMENT_3D('',#21796,#17846,#17847);
#15993=AXIS2_PLACEMENT_3D('',#21808,#17848,#17849);
#15994=AXIS2_PLACEMENT_3D('',#21809,#17850,#17851);
#15995=AXIS2_PLACEMENT_3D('',#21817,#17855,#17856);
#15996=AXIS2_PLACEMENT_3D('',#21819,#17857,#17858);
#15997=AXIS2_PLACEMENT_3D('',#21823,#17860,#17861);
#15998=AXIS2_PLACEMENT_3D('',#21825,#17862,#17863);
#15999=AXIS2_PLACEMENT_3D('',#21830,#17866,#17867);
#16000=AXIS2_PLACEMENT_3D('',#21832,#17868,#17869);
#16001=AXIS2_PLACEMENT_3D('',#21882,#17895,#17896);
#16002=AXIS2_PLACEMENT_3D('',#21886,#17898,#17899);
#16003=AXIS2_PLACEMENT_3D('',#21887,#17900,#17901);
#16004=AXIS2_PLACEMENT_3D('',#21890,#17903,#17904);
#16005=AXIS2_PLACEMENT_3D('',#21945,#17905,#17906);
#16006=AXIS2_PLACEMENT_3D('',#21957,#17908,#17909);
#16007=AXIS2_PLACEMENT_3D('',#22004,#17910,#17911);
#16008=AXIS2_PLACEMENT_3D('',#22005,#17912,#17913);
#16009=AXIS2_PLACEMENT_3D('',#22009,#17915,#17916);
#16010=AXIS2_PLACEMENT_3D('',#22010,#17917,#17918);
#16011=AXIS2_PLACEMENT_3D('',#22013,#17920,#17921);
#16012=AXIS2_PLACEMENT_3D('',#22014,#17922,#17923);
#16013=AXIS2_PLACEMENT_3D('',#22026,#17925,#17926);
#16014=AXIS2_PLACEMENT_3D('',#22027,#17927,#17928);
#16015=AXIS2_PLACEMENT_3D('',#22038,#17929,#17930);
#16016=AXIS2_PLACEMENT_3D('',#22042,#17932,#17933);
#16017=AXIS2_PLACEMENT_3D('',#22043,#17934,#17935);
#16018=AXIS2_PLACEMENT_3D('',#22046,#17937,#17938);
#16019=AXIS2_PLACEMENT_3D('',#22047,#17939,#17940);
#16020=AXIS2_PLACEMENT_3D('',#22049,#17942,#17943);
#16021=AXIS2_PLACEMENT_3D('',#22053,#17945,#17946);
#16022=AXIS2_PLACEMENT_3D('',#22054,#17947,#17948);
#16023=AXIS2_PLACEMENT_3D('',#22057,#17950,#17951);
#16024=AXIS2_PLACEMENT_3D('',#22058,#17952,#17953);
#16025=AXIS2_PLACEMENT_3D('',#22060,#17955,#17956);
#16026=AXIS2_PLACEMENT_3D('',#22064,#17958,#17959);
#16027=AXIS2_PLACEMENT_3D('',#22065,#17960,#17961);
#16028=AXIS2_PLACEMENT_3D('',#22068,#17963,#17964);
#16029=AXIS2_PLACEMENT_3D('',#22069,#17965,#17966);
#16030=AXIS2_PLACEMENT_3D('',#22072,#17968,#17969);
#16031=AXIS2_PLACEMENT_3D('',#22073,#17970,#17971);
#16032=AXIS2_PLACEMENT_3D('',#22077,#17973,#17974);
#16033=AXIS2_PLACEMENT_3D('',#22078,#17975,#17976);
#16034=AXIS2_PLACEMENT_3D('',#22081,#17978,#17979);
#16035=AXIS2_PLACEMENT_3D('',#22082,#17980,#17981);
#16036=AXIS2_PLACEMENT_3D('',#22084,#17983,#17984);
#16037=AXIS2_PLACEMENT_3D('',#22088,#17986,#17987);
#16038=AXIS2_PLACEMENT_3D('',#22089,#17988,#17989);
#16039=AXIS2_PLACEMENT_3D('',#22092,#17991,#17992);
#16040=AXIS2_PLACEMENT_3D('',#22093,#17993,#17994);
#16041=AXIS2_PLACEMENT_3D('',#22096,#17996,#17997);
#16042=AXIS2_PLACEMENT_3D('',#22097,#17998,#17999);
#16043=AXIS2_PLACEMENT_3D('',#22101,#18001,#18002);
#16044=AXIS2_PLACEMENT_3D('',#22102,#18003,#18004);
#16045=AXIS2_PLACEMENT_3D('',#22105,#18006,#18007);
#16046=AXIS2_PLACEMENT_3D('',#22106,#18008,#18009);
#16047=AXIS2_PLACEMENT_3D('',#22108,#18011,#18012);
#16048=AXIS2_PLACEMENT_3D('',#22112,#18014,#18015);
#16049=AXIS2_PLACEMENT_3D('',#22113,#18016,#18017);
#16050=AXIS2_PLACEMENT_3D('',#22116,#18019,#18020);
#16051=AXIS2_PLACEMENT_3D('',#22117,#18021,#18022);
#16052=AXIS2_PLACEMENT_3D('',#22120,#18024,#18025);
#16053=AXIS2_PLACEMENT_3D('',#22121,#18026,#18027);
#16054=AXIS2_PLACEMENT_3D('',#22125,#18029,#18030);
#16055=AXIS2_PLACEMENT_3D('',#22126,#18031,#18032);
#16056=AXIS2_PLACEMENT_3D('',#22129,#18034,#18035);
#16057=AXIS2_PLACEMENT_3D('',#22130,#18036,#18037);
#16058=AXIS2_PLACEMENT_3D('',#22132,#18039,#18040);
#16059=AXIS2_PLACEMENT_3D('',#22136,#18042,#18043);
#16060=AXIS2_PLACEMENT_3D('',#22137,#18044,#18045);
#16061=AXIS2_PLACEMENT_3D('',#22140,#18047,#18048);
#16062=AXIS2_PLACEMENT_3D('',#22141,#18049,#18050);
#16063=AXIS2_PLACEMENT_3D('',#22144,#18052,#18053);
#16064=AXIS2_PLACEMENT_3D('',#22145,#18054,#18055);
#16065=AXIS2_PLACEMENT_3D('',#22149,#18057,#18058);
#16066=AXIS2_PLACEMENT_3D('',#22150,#18059,#18060);
#16067=AXIS2_PLACEMENT_3D('',#22153,#18062,#18063);
#16068=AXIS2_PLACEMENT_3D('',#22154,#18064,#18065);
#16069=AXIS2_PLACEMENT_3D('',#22156,#18067,#18068);
#16070=AXIS2_PLACEMENT_3D('',#22160,#18070,#18071);
#16071=AXIS2_PLACEMENT_3D('',#22161,#18072,#18073);
#16072=AXIS2_PLACEMENT_3D('',#22164,#18075,#18076);
#16073=AXIS2_PLACEMENT_3D('',#22165,#18077,#18078);
#16074=AXIS2_PLACEMENT_3D('',#22167,#18080,#18081);
#16075=AXIS2_PLACEMENT_3D('',#22171,#18083,#18084);
#16076=AXIS2_PLACEMENT_3D('',#22172,#18085,#18086);
#16077=AXIS2_PLACEMENT_3D('',#22175,#18088,#18089);
#16078=AXIS2_PLACEMENT_3D('',#22176,#18090,#18091);
#16079=AXIS2_PLACEMENT_3D('',#22178,#18093,#18094);
#16080=AXIS2_PLACEMENT_3D('',#22182,#18096,#18097);
#16081=AXIS2_PLACEMENT_3D('',#22183,#18098,#18099);
#16082=AXIS2_PLACEMENT_3D('',#22187,#18102,#18103);
#16083=AXIS2_PLACEMENT_3D('',#22188,#18104,#18105);
#16084=AXIS2_PLACEMENT_3D('',#22190,#18107,#18108);
#16085=AXIS2_PLACEMENT_3D('',#22192,#18109,#18110);
#16086=AXIS2_PLACEMENT_3D('',#22195,#18112,#18113);
#16087=AXIS2_PLACEMENT_3D('',#22196,#18114,#18115);
#16088=AXIS2_PLACEMENT_3D('',#22199,#18117,#18118);
#16089=AXIS2_PLACEMENT_3D('',#22200,#18119,#18120);
#16090=AXIS2_PLACEMENT_3D('',#22202,#18121,#18122);
#16091=AXIS2_PLACEMENT_3D('',#22205,#18124,#18125);
#16092=AXIS2_PLACEMENT_3D('',#22206,#18126,#18127);
#16093=AXIS2_PLACEMENT_3D('',#22209,#18129,#18130);
#16094=AXIS2_PLACEMENT_3D('',#22210,#18131,#18132);
#16095=AXIS2_PLACEMENT_3D('',#22212,#18133,#18134);
#16096=AXIS2_PLACEMENT_3D('',#22215,#18136,#18137);
#16097=AXIS2_PLACEMENT_3D('',#22216,#18138,#18139);
#16098=AXIS2_PLACEMENT_3D('',#22219,#18141,#18142);
#16099=AXIS2_PLACEMENT_3D('',#22220,#18143,#18144);
#16100=AXIS2_PLACEMENT_3D('',#22222,#18145,#18146);
#16101=AXIS2_PLACEMENT_3D('',#22225,#18148,#18149);
#16102=AXIS2_PLACEMENT_3D('',#22226,#18150,#18151);
#16103=AXIS2_PLACEMENT_3D('',#22229,#18153,#18154);
#16104=AXIS2_PLACEMENT_3D('',#22230,#18155,#18156);
#16105=AXIS2_PLACEMENT_3D('',#22234,#18159,#18160);
#16106=AXIS2_PLACEMENT_3D('',#22236,#18162,#18163);
#16107=AXIS2_PLACEMENT_3D('',#22240,#18166,#18167);
#16108=AXIS2_PLACEMENT_3D('',#22244,#18170,#18171);
#16109=AXIS2_PLACEMENT_3D('',#22246,#18173,#18174);
#16110=AXIS2_PLACEMENT_3D('',#22248,#18175,#18176);
#16111=AXIS2_PLACEMENT_3D('',#22259,#18182,#18183);
#16112=AXIS2_PLACEMENT_3D('',#22261,#18184,#18185);
#16113=AXIS2_PLACEMENT_3D('',#22262,#18186,#18187);
#16114=AXIS2_PLACEMENT_3D('',#22268,#18191,#18192);
#16115=AXIS2_PLACEMENT_3D('',#22272,#18195,#18196);
#16116=AXIS2_PLACEMENT_3D('',#22277,#18200,#18201);
#16117=AXIS2_PLACEMENT_3D('',#22278,#18202,#18203);
#16118=AXIS2_PLACEMENT_3D('',#22287,#18209,#18210);
#16119=AXIS2_PLACEMENT_3D('',#22290,#18213,#18214);
#16120=AXIS2_PLACEMENT_3D('',#22291,#18215,#18216);
#16121=AXIS2_PLACEMENT_3D('',#22293,#18217,#18218);
#16122=AXIS2_PLACEMENT_3D('',#22295,#18220,#18221);
#16123=AXIS2_PLACEMENT_3D('',#22296,#18222,#18223);
#16124=AXIS2_PLACEMENT_3D('',#22299,#18225,#18226);
#16125=AXIS2_PLACEMENT_3D('',#22300,#18227,#18228);
#16126=AXIS2_PLACEMENT_3D('',#22302,#18229,#18230);
#16127=AXIS2_PLACEMENT_3D('',#22313,#18236,#18237);
#16128=AXIS2_PLACEMENT_3D('',#22314,#18238,#18239);
#16129=AXIS2_PLACEMENT_3D('',#22315,#18240,#18241);
#16130=AXIS2_PLACEMENT_3D('',#22318,#18244,#18245);
#16131=AXIS2_PLACEMENT_3D('',#22321,#18248,#18249);
#16132=AXIS2_PLACEMENT_3D('',#22322,#18250,#18251);
#16133=AXIS2_PLACEMENT_3D('',#22324,#18253,#18254);
#16134=AXIS2_PLACEMENT_3D('',#22326,#18256,#18257);
#16135=AXIS2_PLACEMENT_3D('',#22332,#18261,#18262);
#16136=AXIS2_PLACEMENT_3D('',#22336,#18265,#18266);
#16137=AXIS2_PLACEMENT_3D('',#22340,#18269,#18270);
#16138=AXIS2_PLACEMENT_3D('',#22342,#18272,#18273);
#16139=AXIS2_PLACEMENT_3D('',#22343,#18274,#18275);
#16140=AXIS2_PLACEMENT_3D('',#22349,#18279,#18280);
#16141=AXIS2_PLACEMENT_3D('',#22353,#18283,#18284);
#16142=AXIS2_PLACEMENT_3D('',#22357,#18287,#18288);
#16143=AXIS2_PLACEMENT_3D('',#22359,#18290,#18291);
#16144=AXIS2_PLACEMENT_3D('',#22360,#18292,#18293);
#16145=AXIS2_PLACEMENT_3D('',#22366,#18297,#18298);
#16146=AXIS2_PLACEMENT_3D('',#22370,#18301,#18302);
#16147=AXIS2_PLACEMENT_3D('',#22374,#18305,#18306);
#16148=AXIS2_PLACEMENT_3D('',#22376,#18308,#18309);
#16149=AXIS2_PLACEMENT_3D('',#22377,#18310,#18311);
#16150=AXIS2_PLACEMENT_3D('',#22383,#18315,#18316);
#16151=AXIS2_PLACEMENT_3D('',#22387,#18319,#18320);
#16152=AXIS2_PLACEMENT_3D('',#22391,#18323,#18324);
#16153=AXIS2_PLACEMENT_3D('',#22393,#18326,#18327);
#16154=AXIS2_PLACEMENT_3D('',#22394,#18328,#18329);
#16155=AXIS2_PLACEMENT_3D('',#22400,#18333,#18334);
#16156=AXIS2_PLACEMENT_3D('',#22404,#18337,#18338);
#16157=AXIS2_PLACEMENT_3D('',#22408,#18341,#18342);
#16158=AXIS2_PLACEMENT_3D('',#22410,#18344,#18345);
#16159=AXIS2_PLACEMENT_3D('',#22411,#18346,#18347);
#16160=AXIS2_PLACEMENT_3D('',#22417,#18351,#18352);
#16161=AXIS2_PLACEMENT_3D('',#22421,#18355,#18356);
#16162=AXIS2_PLACEMENT_3D('',#22425,#18359,#18360);
#16163=AXIS2_PLACEMENT_3D('',#22427,#18362,#18363);
#16164=AXIS2_PLACEMENT_3D('',#22428,#18364,#18365);
#16165=AXIS2_PLACEMENT_3D('',#22431,#18367,#18368);
#16166=AXIS2_PLACEMENT_3D('',#22432,#18369,#18370);
#16167=AXIS2_PLACEMENT_3D('',#22434,#18371,#18372);
#16168=AXIS2_PLACEMENT_3D('',#22435,#18373,#18374);
#16169=AXIS2_PLACEMENT_3D('',#22438,#18376,#18377);
#16170=AXIS2_PLACEMENT_3D('',#22439,#18378,#18379);
#16171=AXIS2_PLACEMENT_3D('',#22441,#18380,#18381);
#16172=AXIS2_PLACEMENT_3D('',#22442,#18382,#18383);
#16173=AXIS2_PLACEMENT_3D('',#22445,#18385,#18386);
#16174=AXIS2_PLACEMENT_3D('',#22446,#18387,#18388);
#16175=AXIS2_PLACEMENT_3D('',#22448,#18389,#18390);
#16176=AXIS2_PLACEMENT_3D('',#22449,#18391,#18392);
#16177=AXIS2_PLACEMENT_3D('',#22492,#18395,#18396);
#16178=AXIS2_PLACEMENT_3D('',#22528,#18397,#18398);
#16179=AXIS2_PLACEMENT_3D('',#22530,#18399,#18400);
#16180=AXIS2_PLACEMENT_3D('',#22531,#18401,#18402);
#16181=AXIS2_PLACEMENT_3D('',#22534,#18404,#18405);
#16182=AXIS2_PLACEMENT_3D('',#22535,#18406,#18407);
#16183=AXIS2_PLACEMENT_3D('',#22537,#18408,#18409);
#16184=AXIS2_PLACEMENT_3D('',#22538,#18410,#18411);
#16185=AXIS2_PLACEMENT_3D('',#22541,#18413,#18414);
#16186=AXIS2_PLACEMENT_3D('',#22542,#18415,#18416);
#16187=AXIS2_PLACEMENT_3D('',#22544,#18417,#18418);
#16188=AXIS2_PLACEMENT_3D('',#22545,#18419,#18420);
#16189=AXIS2_PLACEMENT_3D('',#22547,#18422,#18423);
#16190=AXIS2_PLACEMENT_3D('',#22550,#18425,#18426);
#16191=AXIS2_PLACEMENT_3D('',#22551,#18427,#18428);
#16192=AXIS2_PLACEMENT_3D('',#22553,#18429,#18430);
#16193=AXIS2_PLACEMENT_3D('',#22554,#18431,#18432);
#16194=AXIS2_PLACEMENT_3D('',#22557,#18434,#18435);
#16195=AXIS2_PLACEMENT_3D('',#22558,#18436,#18437);
#16196=AXIS2_PLACEMENT_3D('',#22560,#18438,#18439);
#16197=AXIS2_PLACEMENT_3D('',#22561,#18440,#18441);
#16198=AXIS2_PLACEMENT_3D('',#22564,#18443,#18444);
#16199=AXIS2_PLACEMENT_3D('',#22565,#18445,#18446);
#16200=AXIS2_PLACEMENT_3D('',#22567,#18448,#18449);
#16201=AXIS2_PLACEMENT_3D('',#22568,#18450,#18451);
#16202=AXIS2_PLACEMENT_3D('',#22569,#18452,#18453);
#17288=DIRECTION('axis',(0.,0.,1.));
#17289=DIRECTION('refdir',(1.,0.,0.));
#17290=DIRECTION('center_axis',(0.,0.,-1.));
#17291=DIRECTION('ref_axis',(0.,-1.,0.));
#17292=DIRECTION('',(0.,-1.,0.));
#17293=DIRECTION('',(-1.,0.,0.));
#17294=DIRECTION('',(0.,-1.,0.));
#17295=DIRECTION('',(-1.,0.,0.));
#17296=DIRECTION('center_axis',(0.,1.,0.));
#17297=DIRECTION('ref_axis',(0.,0.,-1.));
#17298=DIRECTION('',(0.,0.,-1.));
#17299=DIRECTION('',(-1.,0.,0.));
#17300=DIRECTION('',(0.,0.,-1.));
#17301=DIRECTION('center_axis',(0.,0.,1.));
#17302=DIRECTION('ref_axis',(0.,1.,0.));
#17303=DIRECTION('',(0.,1.,0.));
#17304=DIRECTION('',(-1.,0.,0.));
#17305=DIRECTION('',(0.,1.,0.));
#17306=DIRECTION('center_axis',(0.,-1.,0.));
#17307=DIRECTION('ref_axis',(0.,0.,1.));
#17308=DIRECTION('',(0.,0.,1.));
#17309=DIRECTION('',(0.,0.,1.));
#17310=DIRECTION('center_axis',(-1.,0.,0.));
#17311=DIRECTION('ref_axis',(0.,0.,1.));
#17312=DIRECTION('center_axis',(0.,0.,-1.));
#17313=DIRECTION('ref_axis',(0.,-1.,0.));
#17314=DIRECTION('',(-1.,0.,0.));
#17315=DIRECTION('',(0.,-1.,0.));
#17316=DIRECTION('',(-1.,0.,0.));
#17317=DIRECTION('',(0.,-1.,0.));
#17318=DIRECTION('center_axis',(-1.,0.,0.));
#17319=DIRECTION('ref_axis',(0.,0.,1.));
#17320=DIRECTION('',(0.,0.,1.));
#17321=DIRECTION('',(0.,0.,-1.));
#17322=DIRECTION('',(0.,1.,0.));
#17323=DIRECTION('',(0.,0.,1.));
#17324=DIRECTION('',(0.,-1.,0.));
#17325=DIRECTION('center_axis',(0.,1.,0.));
#17326=DIRECTION('ref_axis',(0.,0.,-1.));
#17327=DIRECTION('',(0.,0.,-1.));
#17328=DIRECTION('',(-1.,0.,0.));
#17329=DIRECTION('center_axis',(0.,0.,1.));
#17330=DIRECTION('ref_axis',(0.,1.,0.));
#17331=DIRECTION('',(0.,1.,0.));
#17332=DIRECTION('',(-1.,0.,0.));
#17333=DIRECTION('center_axis',(0.,-1.,0.));
#17334=DIRECTION('ref_axis',(0.,0.,1.));
#17335=DIRECTION('',(1.,0.,0.));
#17336=DIRECTION('',(0.,0.,1.));
#17337=DIRECTION('center_axis',(0.,0.,-1.));
#17338=DIRECTION('ref_axis',(0.,-1.,0.));
#17339=DIRECTION('',(0.,-1.,0.));
#17340=DIRECTION('',(-1.,0.,0.));
#17341=DIRECTION('',(0.,-1.,0.));
#17342=DIRECTION('',(-1.,0.,0.));
#17343=DIRECTION('center_axis',(0.,1.,0.));
#17344=DIRECTION('ref_axis',(0.,0.,-1.));
#17345=DIRECTION('',(0.,0.,-1.));
#17346=DIRECTION('',(-1.,0.,0.));
#17347=DIRECTION('',(0.,0.,-1.));
#17348=DIRECTION('center_axis',(0.,0.,1.));
#17349=DIRECTION('ref_axis',(0.,1.,0.));
#17350=DIRECTION('',(0.,1.,0.));
#17351=DIRECTION('',(-1.,0.,0.));
#17352=DIRECTION('',(0.,1.,0.));
#17353=DIRECTION('center_axis',(0.,-1.,0.));
#17354=DIRECTION('ref_axis',(0.,0.,1.));
#17355=DIRECTION('',(0.,0.,1.));
#17356=DIRECTION('',(0.,0.,1.));
#17357=DIRECTION('center_axis',(-1.,0.,0.));
#17358=DIRECTION('ref_axis',(0.,0.,1.));
#17359=DIRECTION('center_axis',(0.,0.,-1.));
#17360=DIRECTION('ref_axis',(0.,-1.,0.));
#17361=DIRECTION('',(0.,-1.,0.));
#17362=DIRECTION('',(-1.,0.,0.));
#17363=DIRECTION('',(0.,-1.,0.));
#17364=DIRECTION('',(-1.,0.,0.));
#17365=DIRECTION('center_axis',(0.,1.,0.));
#17366=DIRECTION('ref_axis',(0.,0.,-1.));
#17367=DIRECTION('',(0.,0.,-1.));
#17368=DIRECTION('',(-1.,0.,0.));
#17369=DIRECTION('',(0.,0.,-1.));
#17370=DIRECTION('center_axis',(0.,0.,1.));
#17371=DIRECTION('ref_axis',(0.,1.,0.));
#17372=DIRECTION('',(0.,1.,0.));
#17373=DIRECTION('',(-1.,0.,0.));
#17374=DIRECTION('',(0.,1.,0.));
#17375=DIRECTION('center_axis',(0.,-1.,0.));
#17376=DIRECTION('ref_axis',(0.,0.,1.));
#17377=DIRECTION('',(0.,0.,1.));
#17378=DIRECTION('',(0.,0.,1.));
#17379=DIRECTION('center_axis',(-1.,0.,0.));
#17380=DIRECTION('ref_axis',(0.,0.,1.));
#17381=DIRECTION('center_axis',(0.,0.,-1.));
#17382=DIRECTION('ref_axis',(0.,-1.,0.));
#17383=DIRECTION('',(0.,-1.,0.));
#17384=DIRECTION('',(-1.,0.,0.));
#17385=DIRECTION('',(0.,-1.,0.));
#17386=DIRECTION('',(-1.,0.,0.));
#17387=DIRECTION('center_axis',(0.,1.,0.));
#17388=DIRECTION('ref_axis',(0.,0.,-1.));
#17389=DIRECTION('',(0.,0.,-1.));
#17390=DIRECTION('',(-1.,0.,0.));
#17391=DIRECTION('',(0.,0.,-1.));
#17392=DIRECTION('center_axis',(0.,0.,1.));
#17393=DIRECTION('ref_axis',(0.,1.,0.));
#17394=DIRECTION('',(0.,1.,0.));
#17395=DIRECTION('',(-1.,0.,0.));
#17396=DIRECTION('',(0.,1.,0.));
#17397=DIRECTION('center_axis',(0.,-1.,0.));
#17398=DIRECTION('ref_axis',(0.,0.,1.));
#17399=DIRECTION('',(0.,0.,1.));
#17400=DIRECTION('',(0.,0.,1.));
#17401=DIRECTION('center_axis',(-1.,0.,0.));
#17402=DIRECTION('ref_axis',(0.,0.,1.));
#17403=DIRECTION('center_axis',(0.,0.,-1.));
#17404=DIRECTION('ref_axis',(0.,-1.,0.));
#17405=DIRECTION('',(1.,0.,0.));
#17406=DIRECTION('',(0.,-1.,0.));
#17407=DIRECTION('',(-1.,0.,0.));
#17408=DIRECTION('',(0.,-1.,0.));
#17409=DIRECTION('center_axis',(0.,1.,0.));
#17410=DIRECTION('ref_axis',(0.,0.,-1.));
#17411=DIRECTION('',(-1.,0.,0.));
#17412=DIRECTION('',(0.,0.,-1.));
#17413=DIRECTION('',(-1.,0.,0.));
#17414=DIRECTION('',(0.,0.,-1.));
#17415=DIRECTION('center_axis',(0.,0.,1.));
#17416=DIRECTION('ref_axis',(0.,1.,0.));
#17417=DIRECTION('',(0.,1.,0.));
#17418=DIRECTION('',(-1.,0.,0.));
#17419=DIRECTION('',(0.,1.,0.));
#17420=DIRECTION('center_axis',(0.,-1.,0.));
#17421=DIRECTION('ref_axis',(0.,0.,1.));
#17422=DIRECTION('',(0.,0.,1.));
#17423=DIRECTION('',(0.,0.,1.));
#17424=DIRECTION('center_axis',(-1.,0.,0.));
#17425=DIRECTION('ref_axis',(0.,0.,1.));
#17426=DIRECTION('',(0.,0.,-1.));
#17427=DIRECTION('',(0.,-1.,0.));
#17428=DIRECTION('center_axis',(0.,1.,0.));
#17429=DIRECTION('ref_axis',(1.,0.,0.));
#17430=DIRECTION('',(-1.,0.,0.));
#17431=DIRECTION('',(0.,0.,-1.));
#17432=DIRECTION('',(1.,0.,0.));
#17433=DIRECTION('',(0.,0.,-1.));
#17434=DIRECTION('center_axis',(0.,0.,1.));
#17435=DIRECTION('ref_axis',(-1.,0.,0.));
#17436=DIRECTION('',(0.,1.,0.));
#17437=DIRECTION('',(1.,0.,0.));
#17438=DIRECTION('',(0.,-1.,0.));
#17439=DIRECTION('center_axis',(1.,0.,0.));
#17440=DIRECTION('ref_axis',(0.,0.,-1.));
#17441=DIRECTION('',(0.,-1.,0.));
#17442=DIRECTION('',(0.,0.,1.));
#17443=DIRECTION('',(0.,-1.,0.));
#17444=DIRECTION('',(0.,0.,-1.));
#17445=DIRECTION('',(0.,-1.,0.));
#17446=DIRECTION('',(0.,0.,1.));
#17447=DIRECTION('',(0.,1.,0.));
#17448=DIRECTION('',(0.,0.,-1.));
#17449=DIRECTION('',(0.,1.,0.));
#17450=DIRECTION('',(0.,0.,1.));
#17451=DIRECTION('center_axis',(-1.,0.,0.));
#17452=DIRECTION('ref_axis',(0.,0.,1.));
#17453=DIRECTION('center_axis',(0.,0.,1.));
#17454=DIRECTION('ref_axis',(0.,-1.,0.));
#17455=DIRECTION('',(0.,-1.,0.));
#17456=DIRECTION('',(1.,0.,0.));
#17457=DIRECTION('',(0.,-1.,0.));
#17458=DIRECTION('',(1.,0.,0.));
#17459=DIRECTION('center_axis',(0.,1.,0.));
#17460=DIRECTION('ref_axis',(0.,0.,1.));
#17461=DIRECTION('',(0.,0.,1.));
#17462=DIRECTION('',(1.,0.,0.));
#17463=DIRECTION('',(0.,0.,1.));
#17464=DIRECTION('center_axis',(0.,0.,-1.));
#17465=DIRECTION('ref_axis',(0.,1.,0.));
#17466=DIRECTION('',(0.,1.,0.));
#17467=DIRECTION('',(1.,0.,0.));
#17468=DIRECTION('',(0.,1.,0.));
#17469=DIRECTION('center_axis',(0.,-1.,0.));
#17470=DIRECTION('ref_axis',(0.,0.,-1.));
#17471=DIRECTION('',(0.,0.,-1.));
#17472=DIRECTION('',(0.,0.,-1.));
#17473=DIRECTION('center_axis',(1.,0.,0.));
#17474=DIRECTION('ref_axis',(0.,0.,-1.));
#17475=DIRECTION('center_axis',(0.,0.,-1.));
#17476=DIRECTION('ref_axis',(0.,1.,0.));
#17477=DIRECTION('',(-1.,0.,0.));
#17478=DIRECTION('',(0.,1.,0.));
#17479=DIRECTION('',(1.,0.,0.));
#17480=DIRECTION('',(0.,1.,0.));
#17481=DIRECTION('center_axis',(0.,0.,1.));
#17482=DIRECTION('ref_axis',(0.,-1.,0.));
#17483=DIRECTION('',(0.,-1.,0.));
#17484=DIRECTION('',(1.,0.,0.));
#17485=DIRECTION('',(0.,-1.,0.));
#17486=DIRECTION('',(1.,0.,0.));
#17487=DIRECTION('center_axis',(0.,1.,0.));
#17488=DIRECTION('ref_axis',(0.,0.,1.));
#17489=DIRECTION('',(0.,0.,1.));
#17490=DIRECTION('',(0.,0.,1.));
#17491=DIRECTION('center_axis',(0.,-1.,0.));
#17492=DIRECTION('ref_axis',(0.,0.,-1.));
#17493=DIRECTION('',(1.,0.,0.));
#17494=DIRECTION('',(0.,0.,-1.));
#17495=DIRECTION('',(0.,0.,-1.));
#17496=DIRECTION('center_axis',(1.,0.,0.));
#17497=DIRECTION('ref_axis',(0.,0.,-1.));
#17498=DIRECTION('',(0.,0.,-1.));
#17499=DIRECTION('',(0.,1.,0.));
#17500=DIRECTION('center_axis',(0.,0.,1.));
#17501=DIRECTION('ref_axis',(0.,-1.,0.));
#17502=DIRECTION('',(0.,-1.,0.));
#17503=DIRECTION('',(1.,0.,0.));
#17504=DIRECTION('',(0.,-1.,0.));
#17505=DIRECTION('',(1.,0.,0.));
#17506=DIRECTION('center_axis',(0.,1.,0.));
#17507=DIRECTION('ref_axis',(0.,0.,1.));
#17508=DIRECTION('',(0.,0.,1.));
#17509=DIRECTION('',(1.,0.,0.));
#17510=DIRECTION('',(0.,0.,1.));
#17511=DIRECTION('center_axis',(0.,0.,-1.));
#17512=DIRECTION('ref_axis',(0.,1.,0.));
#17513=DIRECTION('',(0.,1.,0.));
#17514=DIRECTION('',(1.,0.,0.));
#17515=DIRECTION('',(0.,1.,0.));
#17516=DIRECTION('center_axis',(0.,-1.,0.));
#17517=DIRECTION('ref_axis',(0.,0.,-1.));
#17518=DIRECTION('',(0.,0.,-1.));
#17519=DIRECTION('',(0.,0.,-1.));
#17520=DIRECTION('center_axis',(1.,0.,0.));
#17521=DIRECTION('ref_axis',(0.,0.,-1.));
#17522=DIRECTION('center_axis',(0.,0.,1.));
#17523=DIRECTION('ref_axis',(0.,-1.,0.));
#17524=DIRECTION('',(0.,-1.,0.));
#17525=DIRECTION('',(1.,0.,0.));
#17526=DIRECTION('',(0.,-1.,0.));
#17527=DIRECTION('',(1.,0.,0.));
#17528=DIRECTION('center_axis',(0.,1.,0.));
#17529=DIRECTION('ref_axis',(0.,0.,1.));
#17530=DIRECTION('',(0.,0.,1.));
#17531=DIRECTION('',(1.,0.,0.));
#17532=DIRECTION('',(0.,0.,1.));
#17533=DIRECTION('center_axis',(0.,0.,-1.));
#17534=DIRECTION('ref_axis',(0.,1.,0.));
#17535=DIRECTION('',(0.,1.,0.));
#17536=DIRECTION('',(1.,0.,0.));
#17537=DIRECTION('',(0.,1.,0.));
#17538=DIRECTION('center_axis',(0.,-1.,0.));
#17539=DIRECTION('ref_axis',(0.,0.,-1.));
#17540=DIRECTION('',(0.,0.,-1.));
#17541=DIRECTION('',(0.,0.,-1.));
#17542=DIRECTION('center_axis',(1.,0.,0.));
#17543=DIRECTION('ref_axis',(0.,0.,-1.));
#17544=DIRECTION('center_axis',(0.,0.,1.));
#17545=DIRECTION('ref_axis',(0.,-1.,0.));
#17546=DIRECTION('',(0.,-1.,0.));
#17547=DIRECTION('',(1.,0.,0.));
#17548=DIRECTION('',(0.,-1.,0.));
#17549=DIRECTION('',(1.,0.,0.));
#17550=DIRECTION('center_axis',(0.,1.,0.));
#17551=DIRECTION('ref_axis',(0.,0.,1.));
#17552=DIRECTION('',(0.,0.,1.));
#17553=DIRECTION('',(1.,0.,0.));
#17554=DIRECTION('',(0.,0.,1.));
#17555=DIRECTION('center_axis',(0.,0.,-1.));
#17556=DIRECTION('ref_axis',(0.,1.,0.));
#17557=DIRECTION('',(0.,1.,0.));
#17558=DIRECTION('',(1.,0.,0.));
#17559=DIRECTION('',(0.,1.,0.));
#17560=DIRECTION('center_axis',(0.,-1.,0.));
#17561=DIRECTION('ref_axis',(0.,0.,-1.));
#17562=DIRECTION('',(0.,0.,-1.));
#17563=DIRECTION('',(0.,0.,-1.));
#17564=DIRECTION('center_axis',(1.,0.,0.));
#17565=DIRECTION('ref_axis',(0.,0.,-1.));
#17566=DIRECTION('center_axis',(0.,1.,0.));
#17567=DIRECTION('ref_axis',(0.,0.,1.));
#17568=DIRECTION('',(-1.,0.,0.));
#17569=DIRECTION('',(0.,0.,1.));
#17570=DIRECTION('',(1.,0.,0.));
#17571=DIRECTION('',(0.,0.,1.));
#17572=DIRECTION('center_axis',(0.,0.,1.));
#17573=DIRECTION('ref_axis',(0.,-1.,0.));
#17574=DIRECTION('',(0.,-1.,0.));
#17575=DIRECTION('',(0.,-1.,0.));
#17576=DIRECTION('',(1.,0.,0.));
#17577=DIRECTION('center_axis',(0.,0.,-1.));
#17578=DIRECTION('ref_axis',(0.,1.,0.));
#17579=DIRECTION('',(1.,0.,0.));
#17580=DIRECTION('',(0.,1.,0.));
#17581=DIRECTION('',(1.,0.,0.));
#17582=DIRECTION('',(0.,1.,0.));
#17583=DIRECTION('center_axis',(0.,-1.,0.));
#17584=DIRECTION('ref_axis',(0.,0.,-1.));
#17585=DIRECTION('',(0.,0.,-1.));
#17586=DIRECTION('',(0.,0.,-1.));
#17587=DIRECTION('center_axis',(1.,0.,0.));
#17588=DIRECTION('ref_axis',(0.,0.,-1.));
#17589=DIRECTION('',(0.,1.,0.));
#17590=DIRECTION('',(0.,0.,1.));
#17591=DIRECTION('center_axis',(0.,1.,0.));
#17592=DIRECTION('ref_axis',(1.,0.,0.));
#17593=DIRECTION('',(0.,0.,1.));
#17594=DIRECTION('',(1.,0.,0.));
#17595=DIRECTION('',(0.,0.,1.));
#17596=DIRECTION('',(-1.,0.,0.));
#17597=DIRECTION('center_axis',(0.,0.,1.));
#17598=DIRECTION('ref_axis',(1.,0.,0.));
#17599=DIRECTION('',(0.,-1.,0.));
#17600=DIRECTION('',(-1.,0.,0.));
#17601=DIRECTION('',(0.,1.,0.));
#17602=DIRECTION('',(-1.,0.,0.));
#17603=DIRECTION('center_axis',(-1.,0.,0.));
#17604=DIRECTION('ref_axis',(0.,0.,1.));
#17605=DIRECTION('',(0.,-1.,0.));
#17606=DIRECTION('',(0.,0.,-1.));
#17607=DIRECTION('',(0.,-1.,0.));
#17608=DIRECTION('center_axis',(1.,0.,0.));
#17609=DIRECTION('ref_axis',(0.,-1.,0.));
#17610=DIRECTION('center_axis',(1.,0.,0.));
#17611=DIRECTION('ref_axis',(0.,-1.,0.));
#17612=DIRECTION('',(0.,-1.,0.));
#17613=DIRECTION('center_axis',(1.,0.,0.));
#17614=DIRECTION('ref_axis',(0.,-1.,0.));
#17615=DIRECTION('center_axis',(1.,0.,0.));
#17616=DIRECTION('ref_axis',(0.,-1.,0.));
#17617=DIRECTION('',(0.,-1.,0.));
#17618=DIRECTION('',(0.,0.,1.));
#17619=DIRECTION('',(0.,0.,-1.));
#17620=DIRECTION('',(0.,1.,0.));
#17621=DIRECTION('',(0.,0.,1.));
#17622=DIRECTION('',(0.,1.,0.));
#17623=DIRECTION('',(0.,0.,-1.));
#17624=DIRECTION('',(0.,1.,0.));
#17625=DIRECTION('center_axis',(1.,0.,0.));
#17626=DIRECTION('ref_axis',(0.,0.,1.));
#17627=DIRECTION('center_axis',(1.,0.,0.));
#17628=DIRECTION('ref_axis',(0.,-1.,0.));
#17629=DIRECTION('center_axis',(1.,0.,0.));
#17630=DIRECTION('ref_axis',(0.,-1.,0.));
#17631=DIRECTION('center_axis',(0.,1.,0.));
#17632=DIRECTION('ref_axis',(1.,0.,0.));
#17633=DIRECTION('center_axis',(0.,-1.,0.));
#17634=DIRECTION('ref_axis',(1.,0.,0.));
#17635=DIRECTION('',(0.,1.,0.));
#17636=DIRECTION('center_axis',(0.,-1.,0.));
#17637=DIRECTION('ref_axis',(1.,0.,0.));
#17638=DIRECTION('',(0.,1.,0.));
#17639=DIRECTION('center_axis',(0.,1.,0.));
#17640=DIRECTION('ref_axis',(1.,0.,0.));
#17641=DIRECTION('center_axis',(0.,-1.,0.));
#17642=DIRECTION('ref_axis',(1.,0.,0.));
#17643=DIRECTION('',(0.,1.,0.));
#17644=DIRECTION('center_axis',(0.,-1.,0.));
#17645=DIRECTION('ref_axis',(1.,0.,0.));
#17646=DIRECTION('center_axis',(1.,0.,0.));
#17647=DIRECTION('ref_axis',(0.,0.,-1.));
#17648=DIRECTION('',(0.,0.,-1.));
#17649=DIRECTION('',(0.,1.,0.));
#17650=DIRECTION('',(0.,0.,-1.));
#17651=DIRECTION('center_axis',(0.,0.,1.));
#17652=DIRECTION('ref_axis',(1.,0.,0.));
#17653=DIRECTION('',(1.,0.,0.));
#17654=DIRECTION('',(0.,1.,0.));
#17655=DIRECTION('',(1.,0.,0.));
#17656=DIRECTION('center_axis',(-1.,0.,0.));
#17657=DIRECTION('ref_axis',(0.,0.,1.));
#17658=DIRECTION('',(0.,0.,1.));
#17659=DIRECTION('',(0.,1.,0.));
#17660=DIRECTION('',(0.,0.,1.));
#17661=DIRECTION('center_axis',(0.,1.,0.));
#17662=DIRECTION('ref_axis',(1.,0.,0.));
#17663=DIRECTION('center_axis',(0.,-1.,0.));
#17664=DIRECTION('ref_axis',(1.,0.,0.));
#17665=DIRECTION('center_axis',(0.,-1.,0.));
#17666=DIRECTION('ref_axis',(1.,0.,0.));
#17667=DIRECTION('center_axis',(0.,1.,0.));
#17668=DIRECTION('ref_axis',(1.,0.,0.));
#17669=DIRECTION('center_axis',(-1.,0.,0.));
#17670=DIRECTION('ref_axis',(0.,0.,-1.));
#17671=DIRECTION('',(0.,0.,-1.));
#17672=DIRECTION('',(0.,-1.,0.));
#17673=DIRECTION('',(0.,0.,-1.));
#17674=DIRECTION('',(0.,-1.,0.));
#17675=DIRECTION('center_axis',(0.,0.,1.));
#17676=DIRECTION('ref_axis',(-1.,0.,0.));
#17677=DIRECTION('',(-1.,0.,0.));
#17678=DIRECTION('',(0.,-1.,0.));
#17679=DIRECTION('',(-1.,0.,0.));
#17680=DIRECTION('center_axis',(1.,0.,0.));
#17681=DIRECTION('ref_axis',(0.,0.,1.));
#17682=DIRECTION('',(0.,0.,1.));
#17683=DIRECTION('',(0.,-1.,0.));
#17684=DIRECTION('',(0.,0.,1.));
#17685=DIRECTION('center_axis',(0.,1.,0.));
#17686=DIRECTION('ref_axis',(1.,0.,0.));
#17687=DIRECTION('center_axis',(0.,1.,0.));
#17688=DIRECTION('ref_axis',(1.,0.,0.));
#17689=DIRECTION('center_axis',(0.,1.,0.));
#17690=DIRECTION('ref_axis',(1.,0.,0.));
#17691=DIRECTION('center_axis',(0.,1.,0.));
#17692=DIRECTION('ref_axis',(1.,0.,0.));
#17693=DIRECTION('center_axis',(0.,1.,0.));
#17694=DIRECTION('ref_axis',(0.,0.,1.));
#17695=DIRECTION('center_axis',(0.,-1.,0.));
#17696=DIRECTION('ref_axis',(1.,0.,0.));
#17697=DIRECTION('center_axis',(0.,-1.,0.));
#17698=DIRECTION('ref_axis',(1.,0.,0.));
#17699=DIRECTION('center_axis',(0.,-1.,0.));
#17700=DIRECTION('ref_axis',(1.,0.,0.));
#17701=DIRECTION('',(0.,0.,1.));
#17702=DIRECTION('center_axis',(0.,-1.,0.));
#17703=DIRECTION('ref_axis',(-0.707106781186548,0.,0.707106781186548));
#17704=DIRECTION('',(1.,0.,0.));
#17705=DIRECTION('center_axis',(0.,-1.,0.));
#17706=DIRECTION('ref_axis',(0.707106781186548,0.,0.707106781186548));
#17707=DIRECTION('',(-1.,0.,0.));
#17708=DIRECTION('',(0.,0.,-1.));
#17709=DIRECTION('center_axis',(0.,-1.,0.));
#17710=DIRECTION('ref_axis',(1.,0.,0.));
#17711=DIRECTION('center_axis',(0.,-1.,0.));
#17712=DIRECTION('ref_axis',(1.,0.,0.));
#17713=DIRECTION('center_axis',(0.,-1.,0.));
#17714=DIRECTION('ref_axis',(1.,0.,0.));
#17715=DIRECTION('center_axis',(0.,-1.,0.));
#17716=DIRECTION('ref_axis',(-1.,0.,0.));
#17717=DIRECTION('center_axis',(0.,-1.,0.));
#17718=DIRECTION('ref_axis',(-1.,0.,0.));
#17719=DIRECTION('center_axis',(0.,1.,0.));
#17720=DIRECTION('ref_axis',(-1.,0.,0.));
#17721=DIRECTION('center_axis',(0.,-1.,0.));
#17722=DIRECTION('ref_axis',(-1.,0.,0.));
#17723=DIRECTION('center_axis',(0.,-1.,0.));
#17724=DIRECTION('ref_axis',(-1.,0.,0.));
#17725=DIRECTION('center_axis',(0.707106781186548,-0.707106781186548,0.));
#17726=DIRECTION('ref_axis',(0.707104368765779,0.707104368765779,-0.00261215326844819));
#17727=DIRECTION('center_axis',(0.,1.,0.));
#17728=DIRECTION('ref_axis',(-1.,0.,0.));
#17729=DIRECTION('center_axis',(-0.707106781186548,0.707106781186548,0.));
#17730=DIRECTION('ref_axis',(0.,0.,1.));
#17731=DIRECTION('',(0.,0.,-1.));
#17732=DIRECTION('center_axis',(-0.707106781186548,0.707106781186548,0.));
#17733=DIRECTION('ref_axis',(0.707104368771539,0.707104368771539,0.0026121501499));
#17734=DIRECTION('',(0.,0.,1.));
#17735=DIRECTION('center_axis',(0.,-1.,0.));
#17736=DIRECTION('ref_axis',(1.,0.,0.));
#17737=DIRECTION('center_axis',(0.,-1.,0.));
#17738=DIRECTION('ref_axis',(1.,0.,0.));
#17739=DIRECTION('center_axis',(0.,1.,0.));
#17740=DIRECTION('ref_axis',(1.,0.,0.));
#17741=DIRECTION('center_axis',(0.,-1.,0.));
#17742=DIRECTION('ref_axis',(1.,0.,0.));
#17743=DIRECTION('center_axis',(0.,-1.,0.));
#17744=DIRECTION('ref_axis',(1.,0.,0.));
#17745=DIRECTION('center_axis',(0.,1.,0.));
#17746=DIRECTION('ref_axis',(1.,0.,0.));
#17747=DIRECTION('center_axis',(0.,-1.,0.));
#17748=DIRECTION('ref_axis',(-1.,0.,0.));
#17749=DIRECTION('center_axis',(0.,-1.,0.));
#17750=DIRECTION('ref_axis',(-1.,0.,0.));
#17751=DIRECTION('center_axis',(-0.707106781186948,-0.707106781186147,-3.20702973920932E-12));
#17752=DIRECTION('ref_axis',(0.707104368780728,-0.707104368781518,-0.00261214496127044));
#17753=DIRECTION('center_axis',(0.,1.,0.));
#17754=DIRECTION('ref_axis',(-1.,0.,0.));
#17755=DIRECTION('center_axis',(0.707106781186548,0.707106781186548,0.));
#17756=DIRECTION('ref_axis',(0.,0.,-1.));
#17757=DIRECTION('',(0.,0.,1.));
#17758=DIRECTION('center_axis',(0.707106781186948,0.707106781186147,-3.20702973916201E-12));
#17759=DIRECTION('ref_axis',(0.707104368789339,-0.707104368790129,0.00261214029942537));
#17760=DIRECTION('',(0.,0.,-1.));
#17761=DIRECTION('center_axis',(0.,-1.,0.));
#17762=DIRECTION('ref_axis',(1.,0.,0.));
#17763=DIRECTION('center_axis',(0.,1.,0.));
#17764=DIRECTION('ref_axis',(1.,0.,0.));
#17765=DIRECTION('center_axis',(0.,-1.,0.));
#17766=DIRECTION('ref_axis',(1.,0.,0.));
#17767=DIRECTION('center_axis',(0.,-1.,0.));
#17768=DIRECTION('ref_axis',(1.,0.,0.));
#17769=DIRECTION('center_axis',(0.,1.,0.));
#17770=DIRECTION('ref_axis',(1.,0.,0.));
#17771=DIRECTION('center_axis',(0.,-1.,0.));
#17772=DIRECTION('ref_axis',(1.,0.,0.));
#17773=DIRECTION('center_axis',(0.,-1.,0.));
#17774=DIRECTION('ref_axis',(1.,0.,0.));
#17775=DIRECTION('center_axis',(0.,1.,0.));
#17776=DIRECTION('ref_axis',(1.,0.,0.));
#17777=DIRECTION('center_axis',(0.,-1.,0.));
#17778=DIRECTION('ref_axis',(1.,0.,0.));
#17779=DIRECTION('center_axis',(0.,-1.,0.));
#17780=DIRECTION('ref_axis',(1.,0.,0.));
#17781=DIRECTION('center_axis',(0.,1.,0.));
#17782=DIRECTION('ref_axis',(1.,0.,0.));
#17783=DIRECTION('center_axis',(0.,-1.,0.));
#17784=DIRECTION('ref_axis',(1.,0.,0.));
#17785=DIRECTION('center_axis',(0.,-1.,0.));
#17786=DIRECTION('ref_axis',(-1.,0.,0.));
#17787=DIRECTION('center_axis',(0.,1.,0.));
#17788=DIRECTION('ref_axis',(-1.,0.,0.));
#17789=DIRECTION('center_axis',(0.,-1.,0.));
#17790=DIRECTION('ref_axis',(-1.,0.,0.));
#17791=DIRECTION('center_axis',(0.,1.,0.));
#17792=DIRECTION('ref_axis',(1.,0.,0.));
#17793=DIRECTION('',(0.,1.,0.));
#17794=DIRECTION('',(0.,1.,0.));
#17795=DIRECTION('center_axis',(0.,1.,0.));
#17796=DIRECTION('ref_axis',(1.,0.,0.));
#17797=DIRECTION('',(0.,1.,0.));
#17798=DIRECTION('center_axis',(0.,1.,0.));
#17799=DIRECTION('ref_axis',(1.,0.,0.));
#17800=DIRECTION('',(0.,-1.,0.));
#17801=DIRECTION('center_axis',(0.,1.,0.));
#17802=DIRECTION('ref_axis',(1.,0.,0.));
#17803=DIRECTION('',(0.,-1.,0.));
#17804=DIRECTION('center_axis',(0.,1.,0.));
#17805=DIRECTION('ref_axis',(-0.991227900682635,0.,0.132163720091018));
#17806=DIRECTION('',(0.,1.,0.));
#17807=DIRECTION('center_axis',(0.,1.,0.));
#17808=DIRECTION('ref_axis',(1.,0.,0.));
#17809=DIRECTION('',(0.,1.,0.));
#17810=DIRECTION('center_axis',(0.,1.,0.));
#17811=DIRECTION('ref_axis',(1.,0.,0.));
#17812=DIRECTION('center_axis',(0.,-1.,0.));
#17813=DIRECTION('ref_axis',(0.,0.,1.));
#17814=DIRECTION('center_axis',(0.,-1.,0.));
#17815=DIRECTION('ref_axis',(-1.,0.,0.));
#17816=DIRECTION('center_axis',(0.,-1.,0.));
#17817=DIRECTION('ref_axis',(-1.,0.,0.));
#17818=DIRECTION('center_axis',(0.,-1.,0.));
#17819=DIRECTION('ref_axis',(-1.,0.,0.));
#17820=DIRECTION('center_axis',(0.,-1.,0.));
#17821=DIRECTION('ref_axis',(-1.,0.,0.));
#17822=DIRECTION('center_axis',(0.,0.,1.));
#17823=DIRECTION('ref_axis',(1.,0.,0.));
#17824=DIRECTION('',(0.,0.,1.));
#17825=DIRECTION('center_axis',(0.,0.,1.));
#17826=DIRECTION('ref_axis',(1.,0.,0.));
#17827=DIRECTION('center_axis',(0.,0.,1.));
#17828=DIRECTION('ref_axis',(1.,0.,0.));
#17829=DIRECTION('',(-0.707106781186545,-8.6595605623549E-17,0.70710678118655));
#17830=DIRECTION('center_axis',(0.,0.,-1.));
#17831=DIRECTION('ref_axis',(1.,0.,0.));
#17832=DIRECTION('center_axis',(0.,0.,1.));
#17833=DIRECTION('ref_axis',(0.,-1.,0.));
#17834=DIRECTION('',(-1.04972719113862E-16,0.857167300702115,0.515038074910049));
#17835=DIRECTION('center_axis',(0.,0.,1.));
#17836=DIRECTION('ref_axis',(1.,0.,0.));
#17837=DIRECTION('center_axis',(0.,0.,1.));
#17838=DIRECTION('ref_axis',(0.,-1.,0.));
#17839=DIRECTION('',(0.,0.,1.));
#17840=DIRECTION('',(0.,0.,1.));
#17841=DIRECTION('center_axis',(0.,0.,1.));
#17842=DIRECTION('ref_axis',(1.,0.,0.));
#17843=DIRECTION('center_axis',(0.,0.,1.));
#17844=DIRECTION('ref_axis',(0.,-1.,0.));
#17845=DIRECTION('',(-8.65956056235501E-17,0.707106781186554,0.707106781186541));
#17846=DIRECTION('center_axis',(0.,0.,-1.));
#17847=DIRECTION('ref_axis',(0.,-1.,0.));
#17848=DIRECTION('center_axis',(0.,0.,-1.));
#17849=DIRECTION('ref_axis',(0.,-1.,0.));
#17850=DIRECTION('center_axis',(0.,0.,1.));
#17851=DIRECTION('ref_axis',(1.,0.,0.));
#17852=DIRECTION('',(0.,1.,0.));
#17853=DIRECTION('',(-1.,0.,0.));
#17854=DIRECTION('',(0.,-1.,0.));
#17855=DIRECTION('center_axis',(0.,0.,-1.));
#17856=DIRECTION('ref_axis',(0.,-1.,0.));
#17857=DIRECTION('center_axis',(0.,0.,-1.));
#17858=DIRECTION('ref_axis',(0.,-1.,0.));
#17859=DIRECTION('',(0.,-1.,0.));
#17860=DIRECTION('center_axis',(0.,0.,-1.));
#17861=DIRECTION('ref_axis',(0.,-1.,0.));
#17862=DIRECTION('center_axis',(0.,0.,-1.));
#17863=DIRECTION('ref_axis',(0.,-1.,0.));
#17864=DIRECTION('',(0.,-1.,0.));
#17865=DIRECTION('',(0.,1.,0.));
#17866=DIRECTION('center_axis',(0.,0.,-1.));
#17867=DIRECTION('ref_axis',(0.,-1.,0.));
#17868=DIRECTION('center_axis',(0.,0.,-1.));
#17869=DIRECTION('ref_axis',(0.,-1.,0.));
#17870=DIRECTION('',(0.,1.,0.));
#17871=DIRECTION('',(-1.,0.,0.));
#17872=DIRECTION('',(0.,1.,0.));
#17873=DIRECTION('',(1.,0.,0.));
#17874=DIRECTION('',(0.,-1.,0.));
#17875=DIRECTION('',(-1.,0.,0.));
#17876=DIRECTION('',(0.,1.,0.));
#17877=DIRECTION('',(1.,0.,0.));
#17878=DIRECTION('',(0.,-1.,0.));
#17879=DIRECTION('',(-1.,0.,0.));
#17880=DIRECTION('',(0.,1.,0.));
#17881=DIRECTION('',(1.,0.,0.));
#17882=DIRECTION('',(0.,-1.,0.));
#17883=DIRECTION('',(-1.,0.,0.));
#17884=DIRECTION('',(0.,1.,0.));
#17885=DIRECTION('',(1.,0.,0.));
#17886=DIRECTION('',(0.,-1.,0.));
#17887=DIRECTION('',(-1.,0.,0.));
#17888=DIRECTION('',(0.,1.,0.));
#17889=DIRECTION('',(1.,0.,0.));
#17890=DIRECTION('',(0.,-1.,0.));
#17891=DIRECTION('',(-1.,0.,0.));
#17892=DIRECTION('',(0.,1.,0.));
#17893=DIRECTION('',(1.,0.,0.));
#17894=DIRECTION('',(0.,-1.,0.));
#17895=DIRECTION('center_axis',(0.,0.,1.));
#17896=DIRECTION('ref_axis',(0.,-1.,0.));
#17897=DIRECTION('',(-1.04972719113862E-16,0.857167300702115,0.515038074910049));
#17898=DIRECTION('center_axis',(0.,0.,1.));
#17899=DIRECTION('ref_axis',(1.,0.,0.));
#17900=DIRECTION('center_axis',(0.,0.,1.));
#17901=DIRECTION('ref_axis',(0.,-1.,0.));
#17902=DIRECTION('',(0.,0.,1.));
#17903=DIRECTION('center_axis',(0.,0.,1.));
#17904=DIRECTION('ref_axis',(1.,0.,0.));
#17905=DIRECTION('center_axis',(0.,0.,1.));
#17906=DIRECTION('ref_axis',(0.,-1.,0.));
#17907=DIRECTION('',(-8.65956056235503E-17,0.707106781186555,0.70710678118654));
#17908=DIRECTION('center_axis',(0.,-1.,0.));
#17909=DIRECTION('ref_axis',(-0.707106781186548,0.,0.707106781186548));
#17910=DIRECTION('center_axis',(0.,1.,0.));
#17911=DIRECTION('ref_axis',(-0.707106781186548,0.,0.707106781186548));
#17912=DIRECTION('center_axis',(0.,0.,1.));
#17913=DIRECTION('ref_axis',(0.,-1.,0.));
#17914=DIRECTION('',(-1.04972719113862E-16,0.857167300702115,0.515038074910049));
#17915=DIRECTION('center_axis',(0.,0.,1.));
#17916=DIRECTION('ref_axis',(1.,0.,0.));
#17917=DIRECTION('center_axis',(0.,0.,1.));
#17918=DIRECTION('ref_axis',(0.,-1.,0.));
#17919=DIRECTION('',(0.,0.,1.));
#17920=DIRECTION('center_axis',(0.,0.,1.));
#17921=DIRECTION('ref_axis',(1.,0.,0.));
#17922=DIRECTION('center_axis',(0.,0.,1.));
#17923=DIRECTION('ref_axis',(0.,-1.,0.));
#17924=DIRECTION('',(-8.65956056235501E-17,0.707106781186554,0.707106781186541));
#17925=DIRECTION('center_axis',(0.,1.,0.));
#17926=DIRECTION('ref_axis',(0.707106781186548,0.,0.707106781186548));
#17927=DIRECTION('center_axis',(0.,1.,0.));
#17928=DIRECTION('ref_axis',(0.707106781186548,0.,0.707106781186548));
#17929=DIRECTION('center_axis',(0.,0.,1.));
#17930=DIRECTION('ref_axis',(0.,-1.,0.));
#17931=DIRECTION('',(-1.04972719113862E-16,0.857167300702115,0.515038074910049));
#17932=DIRECTION('center_axis',(0.,0.,1.));
#17933=DIRECTION('ref_axis',(1.,0.,0.));
#17934=DIRECTION('center_axis',(0.,0.,1.));
#17935=DIRECTION('ref_axis',(0.,-1.,0.));
#17936=DIRECTION('',(0.,0.,1.));
#17937=DIRECTION('center_axis',(0.,0.,1.));
#17938=DIRECTION('ref_axis',(1.,0.,0.));
#17939=DIRECTION('center_axis',(0.,0.,1.));
#17940=DIRECTION('ref_axis',(0.,-1.,0.));
#17941=DIRECTION('',(-8.65956056235503E-17,0.707106781186555,0.70710678118654));
#17942=DIRECTION('center_axis',(0.,1.,0.));
#17943=DIRECTION('ref_axis',(-1.,0.,0.));
#17944=DIRECTION('',(0.85716730070211,0.515038074910058,-1.04972719113862E-16));
#17945=DIRECTION('center_axis',(0.,1.,0.));
#17946=DIRECTION('ref_axis',(1.,0.,0.));
#17947=DIRECTION('center_axis',(0.,1.,0.));
#17948=DIRECTION('ref_axis',(-1.,0.,0.));
#17949=DIRECTION('',(0.,1.,0.));
#17950=DIRECTION('center_axis',(0.,1.,0.));
#17951=DIRECTION('ref_axis',(1.,0.,0.));
#17952=DIRECTION('center_axis',(0.,1.,0.));
#17953=DIRECTION('ref_axis',(-1.,0.,0.));
#17954=DIRECTION('',(0.707106781186544,0.707106781186551,-8.6595605623549E-17));
#17955=DIRECTION('center_axis',(0.,-1.,0.));
#17956=DIRECTION('ref_axis',(1.,0.,0.));
#17957=DIRECTION('',(-0.85716730070211,-0.515038074910058,-1.04972719113862E-16));
#17958=DIRECTION('center_axis',(0.,-1.,0.));
#17959=DIRECTION('ref_axis',(1.,0.,0.));
#17960=DIRECTION('center_axis',(0.,-1.,0.));
#17961=DIRECTION('ref_axis',(1.,0.,0.));
#17962=DIRECTION('',(0.,-1.,0.));
#17963=DIRECTION('center_axis',(0.,-1.,0.));
#17964=DIRECTION('ref_axis',(1.,0.,0.));
#17965=DIRECTION('center_axis',(0.,-1.,0.));
#17966=DIRECTION('ref_axis',(1.,0.,0.));
#17967=DIRECTION('',(-0.707106781186546,-0.707106781186549,-8.65956056235491E-17));
#17968=DIRECTION('center_axis',(0.,1.,0.));
#17969=DIRECTION('ref_axis',(1.,0.,0.));
#17970=DIRECTION('center_axis',(0.,1.,0.));
#17971=DIRECTION('ref_axis',(-1.,0.,0.));
#17972=DIRECTION('',(0.85716730070211,0.515038074910058,-1.04972719113862E-16));
#17973=DIRECTION('center_axis',(0.,1.,0.));
#17974=DIRECTION('ref_axis',(1.,0.,0.));
#17975=DIRECTION('center_axis',(0.,1.,0.));
#17976=DIRECTION('ref_axis',(-1.,0.,0.));
#17977=DIRECTION('',(0.,1.,0.));
#17978=DIRECTION('center_axis',(0.,1.,0.));
#17979=DIRECTION('ref_axis',(1.,0.,0.));
#17980=DIRECTION('center_axis',(0.,1.,0.));
#17981=DIRECTION('ref_axis',(-1.,0.,0.));
#17982=DIRECTION('',(0.707106781186546,0.707106781186549,-8.65956056235491E-17));
#17983=DIRECTION('center_axis',(0.,-1.,0.));
#17984=DIRECTION('ref_axis',(1.,0.,0.));
#17985=DIRECTION('',(-0.85716730070211,-0.515038074910058,-1.04972719113862E-16));
#17986=DIRECTION('center_axis',(0.,-1.,0.));
#17987=DIRECTION('ref_axis',(1.,0.,0.));
#17988=DIRECTION('center_axis',(0.,-1.,0.));
#17989=DIRECTION('ref_axis',(1.,0.,0.));
#17990=DIRECTION('',(0.,-1.,0.));
#17991=DIRECTION('center_axis',(0.,-1.,0.));
#17992=DIRECTION('ref_axis',(1.,0.,0.));
#17993=DIRECTION('center_axis',(0.,-1.,0.));
#17994=DIRECTION('ref_axis',(1.,0.,0.));
#17995=DIRECTION('',(-0.707106781186544,-0.707106781186551,-8.65956056235489E-17));
#17996=DIRECTION('center_axis',(0.,1.,0.));
#17997=DIRECTION('ref_axis',(1.,0.,0.));
#17998=DIRECTION('center_axis',(0.,1.,0.));
#17999=DIRECTION('ref_axis',(-1.,0.,0.));
#18000=DIRECTION('',(0.85716730070211,0.515038074910058,-1.04972719113862E-16));
#18001=DIRECTION('center_axis',(0.,1.,0.));
#18002=DIRECTION('ref_axis',(1.,0.,0.));
#18003=DIRECTION('center_axis',(0.,1.,0.));
#18004=DIRECTION('ref_axis',(-1.,0.,0.));
#18005=DIRECTION('',(0.,1.,0.));
#18006=DIRECTION('center_axis',(0.,1.,0.));
#18007=DIRECTION('ref_axis',(1.,0.,0.));
#18008=DIRECTION('center_axis',(0.,1.,0.));
#18009=DIRECTION('ref_axis',(-1.,0.,0.));
#18010=DIRECTION('',(0.707106781186544,0.707106781186551,-8.65956056235489E-17));
#18011=DIRECTION('center_axis',(0.,-1.,0.));
#18012=DIRECTION('ref_axis',(1.,0.,0.));
#18013=DIRECTION('',(-0.85716730070211,-0.515038074910058,-1.04972719113862E-16));
#18014=DIRECTION('center_axis',(0.,-1.,0.));
#18015=DIRECTION('ref_axis',(1.,0.,0.));
#18016=DIRECTION('center_axis',(0.,-1.,0.));
#18017=DIRECTION('ref_axis',(1.,0.,0.));
#18018=DIRECTION('',(0.,-1.,0.));
#18019=DIRECTION('center_axis',(0.,-1.,0.));
#18020=DIRECTION('ref_axis',(1.,0.,0.));
#18021=DIRECTION('center_axis',(0.,-1.,0.));
#18022=DIRECTION('ref_axis',(1.,0.,0.));
#18023=DIRECTION('',(-0.707106781186544,-0.707106781186551,-8.6595605623549E-17));
#18024=DIRECTION('center_axis',(0.,1.,0.));
#18025=DIRECTION('ref_axis',(1.,0.,0.));
#18026=DIRECTION('center_axis',(0.,1.,0.));
#18027=DIRECTION('ref_axis',(-1.,0.,0.));
#18028=DIRECTION('',(0.85716730070211,0.515038074910058,-1.04972719113862E-16));
#18029=DIRECTION('center_axis',(0.,1.,0.));
#18030=DIRECTION('ref_axis',(1.,0.,0.));
#18031=DIRECTION('center_axis',(0.,1.,0.));
#18032=DIRECTION('ref_axis',(-1.,0.,0.));
#18033=DIRECTION('',(0.,1.,0.));
#18034=DIRECTION('center_axis',(0.,1.,0.));
#18035=DIRECTION('ref_axis',(1.,0.,0.));
#18036=DIRECTION('center_axis',(0.,1.,0.));
#18037=DIRECTION('ref_axis',(-1.,0.,0.));
#18038=DIRECTION('',(0.707106781186544,0.707106781186551,-8.65956056235489E-17));
#18039=DIRECTION('center_axis',(0.,-1.,0.));
#18040=DIRECTION('ref_axis',(1.,0.,0.));
#18041=DIRECTION('',(-0.85716730070211,-0.515038074910058,-1.04972719113862E-16));
#18042=DIRECTION('center_axis',(0.,-1.,0.));
#18043=DIRECTION('ref_axis',(1.,0.,0.));
#18044=DIRECTION('center_axis',(0.,-1.,0.));
#18045=DIRECTION('ref_axis',(1.,0.,0.));
#18046=DIRECTION('',(0.,-1.,0.));
#18047=DIRECTION('center_axis',(0.,-1.,0.));
#18048=DIRECTION('ref_axis',(1.,0.,0.));
#18049=DIRECTION('center_axis',(0.,-1.,0.));
#18050=DIRECTION('ref_axis',(1.,0.,0.));
#18051=DIRECTION('',(-0.707106781186544,-0.707106781186551,-8.6595605623549E-17));
#18052=DIRECTION('center_axis',(0.,1.,0.));
#18053=DIRECTION('ref_axis',(1.,0.,0.));
#18054=DIRECTION('center_axis',(-1.,0.,0.));
#18055=DIRECTION('ref_axis',(0.,-1.,0.));
#18056=DIRECTION('',(-0.515038074910058,0.85716730070211,-1.04972719113862E-16));
#18057=DIRECTION('center_axis',(-1.,0.,0.));
#18058=DIRECTION('ref_axis',(0.,0.,1.));
#18059=DIRECTION('center_axis',(-1.,0.,0.));
#18060=DIRECTION('ref_axis',(0.,-1.,0.));
#18061=DIRECTION('',(-1.,0.,0.));
#18062=DIRECTION('center_axis',(-1.,0.,0.));
#18063=DIRECTION('ref_axis',(0.,0.,1.));
#18064=DIRECTION('center_axis',(-1.,0.,0.));
#18065=DIRECTION('ref_axis',(0.,-1.,0.));
#18066=DIRECTION('',(-0.707106781186546,0.707106781186549,-8.65956056235496E-17));
#18067=DIRECTION('center_axis',(-1.,0.,0.));
#18068=DIRECTION('ref_axis',(0.,-1.,0.));
#18069=DIRECTION('',(-0.515038074910058,0.85716730070211,-1.04972719113862E-16));
#18070=DIRECTION('center_axis',(-1.,0.,0.));
#18071=DIRECTION('ref_axis',(0.,0.,1.));
#18072=DIRECTION('center_axis',(-1.,0.,0.));
#18073=DIRECTION('ref_axis',(0.,-1.,0.));
#18074=DIRECTION('',(-1.,0.,0.));
#18075=DIRECTION('center_axis',(-1.,0.,0.));
#18076=DIRECTION('ref_axis',(0.,0.,1.));
#18077=DIRECTION('center_axis',(-1.,0.,0.));
#18078=DIRECTION('ref_axis',(0.,-1.,0.));
#18079=DIRECTION('',(-0.707106781186548,0.707106781186547,-8.65956056235493E-17));
#18080=DIRECTION('center_axis',(-1.,0.,0.));
#18081=DIRECTION('ref_axis',(0.,-1.,0.));
#18082=DIRECTION('',(-0.515038074910058,0.85716730070211,-1.04972719113862E-16));
#18083=DIRECTION('center_axis',(-1.,0.,0.));
#18084=DIRECTION('ref_axis',(0.,0.,1.));
#18085=DIRECTION('center_axis',(-1.,0.,0.));
#18086=DIRECTION('ref_axis',(0.,-1.,0.));
#18087=DIRECTION('',(-1.,0.,0.));
#18088=DIRECTION('center_axis',(-1.,0.,0.));
#18089=DIRECTION('ref_axis',(0.,0.,1.));
#18090=DIRECTION('center_axis',(-1.,0.,0.));
#18091=DIRECTION('ref_axis',(0.,-1.,0.));
#18092=DIRECTION('',(-0.707106781186546,0.707106781186549,-8.65956056235496E-17));
#18093=DIRECTION('center_axis',(-1.,0.,0.));
#18094=DIRECTION('ref_axis',(0.,-1.,0.));
#18095=DIRECTION('',(-0.515038074910058,0.85716730070211,-1.04972719113862E-16));
#18096=DIRECTION('center_axis',(-1.,0.,0.));
#18097=DIRECTION('ref_axis',(0.,0.,1.));
#18098=DIRECTION('center_axis',(-1.,0.,0.));
#18099=DIRECTION('ref_axis',(0.,-1.,0.));
#18100=DIRECTION('',(-1.,0.,0.));
#18101=DIRECTION('',(-1.,0.,0.));
#18102=DIRECTION('center_axis',(-1.,0.,0.));
#18103=DIRECTION('ref_axis',(0.,0.,1.));
#18104=DIRECTION('center_axis',(-1.,0.,0.));
#18105=DIRECTION('ref_axis',(0.,-1.,0.));
#18106=DIRECTION('',(-0.707106781186548,0.707106781186547,-8.65956056235493E-17));
#18107=DIRECTION('center_axis',(0.,0.,-1.));
#18108=DIRECTION('ref_axis',(0.,1.,0.));
#18109=DIRECTION('center_axis',(0.,0.,-1.));
#18110=DIRECTION('ref_axis',(0.,1.,0.));
#18111=DIRECTION('',(0.,0.,-1.));
#18112=DIRECTION('center_axis',(0.,0.,-1.));
#18113=DIRECTION('ref_axis',(1.,0.,0.));
#18114=DIRECTION('center_axis',(0.,0.,-1.));
#18115=DIRECTION('ref_axis',(0.,1.,0.));
#18116=DIRECTION('',(-8.65956056235492E-17,-0.707106781186547,-0.707106781186548));
#18117=DIRECTION('center_axis',(0.,0.,1.));
#18118=DIRECTION('ref_axis',(0.,1.,0.));
#18119=DIRECTION('center_axis',(0.,0.,-1.));
#18120=DIRECTION('ref_axis',(0.,1.,0.));
#18121=DIRECTION('center_axis',(0.,0.,-1.));
#18122=DIRECTION('ref_axis',(0.,1.,0.));
#18123=DIRECTION('',(0.,0.,-1.));
#18124=DIRECTION('center_axis',(0.,0.,-1.));
#18125=DIRECTION('ref_axis',(1.,0.,0.));
#18126=DIRECTION('center_axis',(0.,0.,-1.));
#18127=DIRECTION('ref_axis',(0.,1.,0.));
#18128=DIRECTION('',(-8.6595605623549E-17,-0.707106781186544,-0.707106781186551));
#18129=DIRECTION('center_axis',(0.,0.,1.));
#18130=DIRECTION('ref_axis',(0.,1.,0.));
#18131=DIRECTION('center_axis',(0.,0.,-1.));
#18132=DIRECTION('ref_axis',(0.,1.,0.));
#18133=DIRECTION('center_axis',(0.,0.,-1.));
#18134=DIRECTION('ref_axis',(0.,1.,0.));
#18135=DIRECTION('',(0.,0.,-1.));
#18136=DIRECTION('center_axis',(0.,0.,-1.));
#18137=DIRECTION('ref_axis',(1.,0.,0.));
#18138=DIRECTION('center_axis',(0.,0.,-1.));
#18139=DIRECTION('ref_axis',(0.,1.,0.));
#18140=DIRECTION('',(-8.65956056235492E-17,-0.707106781186547,-0.707106781186548));
#18141=DIRECTION('center_axis',(0.,0.,1.));
#18142=DIRECTION('ref_axis',(0.,1.,0.));
#18143=DIRECTION('center_axis',(0.,0.,-1.));
#18144=DIRECTION('ref_axis',(0.,1.,0.));
#18145=DIRECTION('center_axis',(0.,0.,-1.));
#18146=DIRECTION('ref_axis',(0.,1.,0.));
#18147=DIRECTION('',(0.,0.,-1.));
#18148=DIRECTION('center_axis',(0.,0.,-1.));
#18149=DIRECTION('ref_axis',(1.,0.,0.));
#18150=DIRECTION('center_axis',(0.,0.,-1.));
#18151=DIRECTION('ref_axis',(0.,1.,0.));
#18152=DIRECTION('',(-8.6595605623549E-17,-0.707106781186544,-0.707106781186551));
#18153=DIRECTION('center_axis',(0.,0.,1.));
#18154=DIRECTION('ref_axis',(0.,1.,0.));
#18155=DIRECTION('center_axis',(-1.,0.,0.));
#18156=DIRECTION('ref_axis',(0.,0.,-1.));
#18157=DIRECTION('',(0.,0.,1.));
#18158=DIRECTION('',(0.,-1.,0.));
#18159=DIRECTION('center_axis',(0.,0.,-1.));
#18160=DIRECTION('ref_axis',(1.,0.,0.));
#18161=DIRECTION('',(-1.,0.,0.));
#18162=DIRECTION('center_axis',(0.,0.,1.));
#18163=DIRECTION('ref_axis',(-1.,0.,0.));
#18164=DIRECTION('',(0.,-1.,0.));
#18165=DIRECTION('',(1.,0.,0.));
#18166=DIRECTION('center_axis',(1.,0.,0.));
#18167=DIRECTION('ref_axis',(0.,0.,1.));
#18168=DIRECTION('',(0.,0.,-1.));
#18169=DIRECTION('',(0.,-1.,0.));
#18170=DIRECTION('center_axis',(0.,0.,-1.));
#18171=DIRECTION('ref_axis',(1.,0.,0.));
#18172=DIRECTION('',(-1.,0.,0.));
#18173=DIRECTION('center_axis',(0.,-1.,0.));
#18174=DIRECTION('ref_axis',(0.,0.,-1.));
#18175=DIRECTION('center_axis',(0.,1.,0.));
#18176=DIRECTION('ref_axis',(-0.707106781186548,0.,-0.707106781186547));
#18177=DIRECTION('',(1.,0.,0.));
#18178=DIRECTION('',(0.,0.,1.));
#18179=DIRECTION('',(1.,0.,0.));
#18180=DIRECTION('',(0.,0.,-1.));
#18181=DIRECTION('',(1.,0.,0.));
#18182=DIRECTION('center_axis',(0.,1.,0.));
#18183=DIRECTION('ref_axis',(0.707106781186549,0.,-0.707106781186546));
#18184=DIRECTION('center_axis',(0.,1.,0.));
#18185=DIRECTION('ref_axis',(0.,0.,1.));
#18186=DIRECTION('center_axis',(0.,0.,-1.));
#18187=DIRECTION('ref_axis',(-1.,0.,0.));
#18188=DIRECTION('',(1.,0.,0.));
#18189=DIRECTION('',(0.,1.,0.));
#18190=DIRECTION('',(1.,0.,0.));
#18191=DIRECTION('center_axis',(0.,1.,0.));
#18192=DIRECTION('ref_axis',(1.,0.,0.));
#18193=DIRECTION('',(0.,0.,-1.));
#18194=DIRECTION('',(-1.,0.,0.));
#18195=DIRECTION('center_axis',(-1.,0.,0.));
#18196=DIRECTION('ref_axis',(0.,0.,1.));
#18197=DIRECTION('',(0.,1.,0.));
#18198=DIRECTION('',(0.,0.,-1.));
#18199=DIRECTION('',(0.,-1.,0.));
#18200=DIRECTION('center_axis',(0.,0.,1.));
#18201=DIRECTION('ref_axis',(1.,0.,0.));
#18202=DIRECTION('center_axis',(1.,0.,0.));
#18203=DIRECTION('ref_axis',(0.,0.,-1.));
#18204=DIRECTION('',(0.,1.,0.));
#18205=DIRECTION('',(0.,0.,1.));
#18206=DIRECTION('',(0.,1.,0.));
#18207=DIRECTION('',(0.,0.,1.));
#18208=DIRECTION('',(0.,-1.,0.));
#18209=DIRECTION('center_axis',(0.,0.,-1.));
#18210=DIRECTION('ref_axis',(-1.,0.,0.));
#18211=DIRECTION('',(1.,0.,0.));
#18212=DIRECTION('',(1.,0.,0.));
#18213=DIRECTION('center_axis',(0.,1.,0.));
#18214=DIRECTION('ref_axis',(1.,0.,0.));
#18215=DIRECTION('center_axis',(0.,1.,0.));
#18216=DIRECTION('ref_axis',(1.,0.,0.));
#18217=DIRECTION('center_axis',(0.,-1.,0.));
#18218=DIRECTION('ref_axis',(1.,0.,0.));
#18219=DIRECTION('',(0.,1.,0.));
#18220=DIRECTION('center_axis',(0.,1.,0.));
#18221=DIRECTION('ref_axis',(1.,0.,0.));
#18222=DIRECTION('center_axis',(0.,1.,0.));
#18223=DIRECTION('ref_axis',(1.,0.,0.));
#18224=DIRECTION('',(0.,1.,0.));
#18225=DIRECTION('center_axis',(0.,-1.,0.));
#18226=DIRECTION('ref_axis',(1.,0.,0.));
#18227=DIRECTION('center_axis',(0.,1.,0.));
#18228=DIRECTION('ref_axis',(0.,0.,1.));
#18229=DIRECTION('center_axis',(0.,-1.,0.));
#18230=DIRECTION('ref_axis',(0.707106781186549,0.,-0.707106781186546));
#18231=DIRECTION('',(-1.,0.,0.));
#18232=DIRECTION('',(0.,0.,1.));
#18233=DIRECTION('',(-1.,0.,0.));
#18234=DIRECTION('',(0.,0.,-1.));
#18235=DIRECTION('',(-1.,0.,0.));
#18236=DIRECTION('center_axis',(0.,-1.,0.));
#18237=DIRECTION('ref_axis',(-0.707106781186548,0.,-0.707106781186547));
#18238=DIRECTION('center_axis',(0.,-1.,0.));
#18239=DIRECTION('ref_axis',(1.,0.,0.));
#18240=DIRECTION('center_axis',(-1.,0.,0.));
#18241=DIRECTION('ref_axis',(0.,0.,1.));
#18242=DIRECTION('',(0.,-1.,0.));
#18243=DIRECTION('',(0.,-1.,0.));
#18244=DIRECTION('center_axis',(1.,0.,0.));
#18245=DIRECTION('ref_axis',(0.,0.,-1.));
#18246=DIRECTION('',(0.,1.,0.));
#18247=DIRECTION('',(0.,1.,0.));
#18248=DIRECTION('center_axis',(0.,0.,1.));
#18249=DIRECTION('ref_axis',(1.,0.,0.));
#18250=DIRECTION('center_axis',(0.,0.,-1.));
#18251=DIRECTION('ref_axis',(-1.,0.,0.));
#18252=DIRECTION('',(0.,1.,0.));
#18253=DIRECTION('center_axis',(0.,0.,-1.));
#18254=DIRECTION('ref_axis',(-1.,0.,0.));
#18255=DIRECTION('',(0.,-1.,0.));
#18256=DIRECTION('center_axis',(0.,-1.,0.));
#18257=DIRECTION('ref_axis',(-1.,0.,0.));
#18258=DIRECTION('',(0.,0.,-1.));
#18259=DIRECTION('',(-1.,0.,0.));
#18260=DIRECTION('',(0.,0.,-1.));
#18261=DIRECTION('center_axis',(1.,0.,0.));
#18262=DIRECTION('ref_axis',(0.,-1.,0.));
#18263=DIRECTION('',(0.,0.,-1.));
#18264=DIRECTION('',(0.,-1.,0.));
#18265=DIRECTION('center_axis',(0.,1.,0.));
#18266=DIRECTION('ref_axis',(1.,0.,0.));
#18267=DIRECTION('',(0.,0.,-1.));
#18268=DIRECTION('',(1.,0.,0.));
#18269=DIRECTION('center_axis',(-1.,0.,0.));
#18270=DIRECTION('ref_axis',(0.,1.,0.));
#18271=DIRECTION('',(0.,1.,0.));
#18272=DIRECTION('center_axis',(0.,0.,-1.));
#18273=DIRECTION('ref_axis',(-1.,0.,0.));
#18274=DIRECTION('center_axis',(0.,-1.,0.));
#18275=DIRECTION('ref_axis',(-1.,0.,0.));
#18276=DIRECTION('',(0.,0.,-1.));
#18277=DIRECTION('',(-1.,0.,0.));
#18278=DIRECTION('',(0.,0.,-1.));
#18279=DIRECTION('center_axis',(1.,0.,0.));
#18280=DIRECTION('ref_axis',(0.,-1.,0.));
#18281=DIRECTION('',(0.,0.,-1.));
#18282=DIRECTION('',(0.,-1.,0.));
#18283=DIRECTION('center_axis',(0.,1.,0.));
#18284=DIRECTION('ref_axis',(1.,0.,0.));
#18285=DIRECTION('',(0.,0.,-1.));
#18286=DIRECTION('',(1.,0.,0.));
#18287=DIRECTION('center_axis',(-1.,0.,0.));
#18288=DIRECTION('ref_axis',(0.,1.,0.));
#18289=DIRECTION('',(0.,1.,0.));
#18290=DIRECTION('center_axis',(0.,0.,-1.));
#18291=DIRECTION('ref_axis',(-1.,0.,0.));
#18292=DIRECTION('center_axis',(0.,-1.,0.));
#18293=DIRECTION('ref_axis',(-1.,0.,0.));
#18294=DIRECTION('',(0.,0.,-1.));
#18295=DIRECTION('',(-1.,0.,0.));
#18296=DIRECTION('',(0.,0.,-1.));
#18297=DIRECTION('center_axis',(1.,0.,0.));
#18298=DIRECTION('ref_axis',(0.,-1.,0.));
#18299=DIRECTION('',(0.,0.,-1.));
#18300=DIRECTION('',(0.,-1.,0.));
#18301=DIRECTION('center_axis',(0.,1.,0.));
#18302=DIRECTION('ref_axis',(1.,0.,0.));
#18303=DIRECTION('',(0.,0.,-1.));
#18304=DIRECTION('',(1.,0.,0.));
#18305=DIRECTION('center_axis',(-1.,0.,0.));
#18306=DIRECTION('ref_axis',(0.,1.,0.));
#18307=DIRECTION('',(0.,1.,0.));
#18308=DIRECTION('center_axis',(0.,0.,-1.));
#18309=DIRECTION('ref_axis',(-1.,0.,0.));
#18310=DIRECTION('center_axis',(0.,-1.,0.));
#18311=DIRECTION('ref_axis',(-1.,0.,0.));
#18312=DIRECTION('',(0.,0.,-1.));
#18313=DIRECTION('',(-1.,0.,0.));
#18314=DIRECTION('',(0.,0.,-1.));
#18315=DIRECTION('center_axis',(1.,0.,0.));
#18316=DIRECTION('ref_axis',(0.,-1.,0.));
#18317=DIRECTION('',(0.,0.,-1.));
#18318=DIRECTION('',(0.,-1.,0.));
#18319=DIRECTION('center_axis',(0.,1.,0.));
#18320=DIRECTION('ref_axis',(1.,0.,0.));
#18321=DIRECTION('',(0.,0.,-1.));
#18322=DIRECTION('',(1.,0.,0.));
#18323=DIRECTION('center_axis',(-1.,0.,0.));
#18324=DIRECTION('ref_axis',(0.,1.,0.));
#18325=DIRECTION('',(0.,1.,0.));
#18326=DIRECTION('center_axis',(0.,0.,-1.));
#18327=DIRECTION('ref_axis',(-1.,0.,0.));
#18328=DIRECTION('center_axis',(0.,-1.,0.));
#18329=DIRECTION('ref_axis',(-1.,0.,0.));
#18330=DIRECTION('',(0.,0.,-1.));
#18331=DIRECTION('',(-1.,0.,0.));
#18332=DIRECTION('',(0.,0.,-1.));
#18333=DIRECTION('center_axis',(1.,0.,0.));
#18334=DIRECTION('ref_axis',(0.,-1.,0.));
#18335=DIRECTION('',(0.,0.,-1.));
#18336=DIRECTION('',(0.,-1.,0.));
#18337=DIRECTION('center_axis',(0.,1.,0.));
#18338=DIRECTION('ref_axis',(1.,0.,0.));
#18339=DIRECTION('',(0.,0.,-1.));
#18340=DIRECTION('',(1.,0.,0.));
#18341=DIRECTION('center_axis',(-1.,0.,0.));
#18342=DIRECTION('ref_axis',(0.,1.,0.));
#18343=DIRECTION('',(0.,1.,0.));
#18344=DIRECTION('center_axis',(0.,0.,-1.));
#18345=DIRECTION('ref_axis',(-1.,0.,0.));
#18346=DIRECTION('center_axis',(0.,-1.,0.));
#18347=DIRECTION('ref_axis',(-1.,0.,0.));
#18348=DIRECTION('',(0.,0.,-1.));
#18349=DIRECTION('',(-1.,0.,0.));
#18350=DIRECTION('',(0.,0.,-1.));
#18351=DIRECTION('center_axis',(1.,0.,0.));
#18352=DIRECTION('ref_axis',(0.,-1.,0.));
#18353=DIRECTION('',(0.,0.,-1.));
#18354=DIRECTION('',(0.,-1.,0.));
#18355=DIRECTION('center_axis',(0.,1.,0.));
#18356=DIRECTION('ref_axis',(1.,0.,0.));
#18357=DIRECTION('',(0.,0.,-1.));
#18358=DIRECTION('',(1.,0.,0.));
#18359=DIRECTION('center_axis',(-1.,0.,0.));
#18360=DIRECTION('ref_axis',(0.,1.,0.));
#18361=DIRECTION('',(0.,1.,0.));
#18362=DIRECTION('center_axis',(0.,0.,-1.));
#18363=DIRECTION('ref_axis',(-1.,0.,0.));
#18364=DIRECTION('center_axis',(-1.,0.,0.));
#18365=DIRECTION('ref_axis',(0.,0.,1.));
#18366=DIRECTION('',(-1.,0.,0.));
#18367=DIRECTION('center_axis',(-1.,0.,0.));
#18368=DIRECTION('ref_axis',(0.,0.,1.));
#18369=DIRECTION('center_axis',(1.,0.,0.));
#18370=DIRECTION('ref_axis',(0.,0.,-1.));
#18371=DIRECTION('center_axis',(-1.,0.,0.));
#18372=DIRECTION('ref_axis',(0.,0.,1.));
#18373=DIRECTION('center_axis',(-1.,0.,0.));
#18374=DIRECTION('ref_axis',(0.,0.,1.));
#18375=DIRECTION('',(-1.,0.,0.));
#18376=DIRECTION('center_axis',(-1.,0.,0.));
#18377=DIRECTION('ref_axis',(0.,0.,1.));
#18378=DIRECTION('center_axis',(-1.,0.,0.));
#18379=DIRECTION('ref_axis',(0.,0.,1.));
#18380=DIRECTION('center_axis',(-1.,0.,0.));
#18381=DIRECTION('ref_axis',(0.,0.,1.));
#18382=DIRECTION('center_axis',(-1.,0.,0.));
#18383=DIRECTION('ref_axis',(0.,0.,1.));
#18384=DIRECTION('',(-1.,0.,0.));
#18385=DIRECTION('center_axis',(-1.,0.,0.));
#18386=DIRECTION('ref_axis',(0.,0.,1.));
#18387=DIRECTION('center_axis',(-1.,0.,0.));
#18388=DIRECTION('ref_axis',(0.,0.,1.));
#18389=DIRECTION('center_axis',(-1.,0.,0.));
#18390=DIRECTION('ref_axis',(0.,0.,1.));
#18391=DIRECTION('center_axis',(-1.,0.,0.));
#18392=DIRECTION('ref_axis',(0.,0.,1.));
#18393=DIRECTION('',(-1.,0.,0.));
#18394=DIRECTION('',(-1.,0.,0.));
#18395=DIRECTION('center_axis',(-1.,0.,0.));
#18396=DIRECTION('ref_axis',(0.,0.,1.));
#18397=DIRECTION('center_axis',(1.,0.,0.));
#18398=DIRECTION('ref_axis',(0.,0.,-1.));
#18399=DIRECTION('center_axis',(-1.,0.,0.));
#18400=DIRECTION('ref_axis',(0.,0.,1.));
#18401=DIRECTION('center_axis',(-1.,0.,0.));
#18402=DIRECTION('ref_axis',(0.,0.,1.));
#18403=DIRECTION('',(-1.,0.,0.));
#18404=DIRECTION('center_axis',(-1.,0.,0.));
#18405=DIRECTION('ref_axis',(0.,0.,1.));
#18406=DIRECTION('center_axis',(1.,0.,0.));
#18407=DIRECTION('ref_axis',(0.,0.,-1.));
#18408=DIRECTION('center_axis',(-1.,0.,0.));
#18409=DIRECTION('ref_axis',(0.,0.,1.));
#18410=DIRECTION('center_axis',(-1.,0.,0.));
#18411=DIRECTION('ref_axis',(0.,0.,1.));
#18412=DIRECTION('',(-1.,0.,0.));
#18413=DIRECTION('center_axis',(-1.,0.,0.));
#18414=DIRECTION('ref_axis',(0.,0.,1.));
#18415=DIRECTION('center_axis',(-1.,0.,0.));
#18416=DIRECTION('ref_axis',(0.,0.,1.));
#18417=DIRECTION('center_axis',(-1.,0.,0.));
#18418=DIRECTION('ref_axis',(0.,0.,1.));
#18419=DIRECTION('center_axis',(-1.,0.,0.));
#18420=DIRECTION('ref_axis',(0.,0.,1.));
#18421=DIRECTION('',(-1.,0.,0.));
#18422=DIRECTION('center_axis',(0.,1.,0.));
#18423=DIRECTION('ref_axis',(0.,0.,1.));
#18424=DIRECTION('',(0.,1.,0.));
#18425=DIRECTION('center_axis',(0.,1.,0.));
#18426=DIRECTION('ref_axis',(1.,0.,0.));
#18427=DIRECTION('center_axis',(0.,1.,0.));
#18428=DIRECTION('ref_axis',(0.,0.,1.));
#18429=DIRECTION('center_axis',(0.,1.,0.));
#18430=DIRECTION('ref_axis',(1.,0.,0.));
#18431=DIRECTION('center_axis',(0.,1.,0.));
#18432=DIRECTION('ref_axis',(0.,0.,1.));
#18433=DIRECTION('',(0.,1.,0.));
#18434=DIRECTION('center_axis',(0.,1.,0.));
#18435=DIRECTION('ref_axis',(1.,0.,0.));
#18436=DIRECTION('center_axis',(0.,1.,0.));
#18437=DIRECTION('ref_axis',(0.,0.,1.));
#18438=DIRECTION('center_axis',(0.,1.,0.));
#18439=DIRECTION('ref_axis',(1.,0.,0.));
#18440=DIRECTION('center_axis',(0.,1.,0.));
#18441=DIRECTION('ref_axis',(0.,0.,1.));
#18442=DIRECTION('',(0.,1.,0.));
#18443=DIRECTION('center_axis',(0.,1.,0.));
#18444=DIRECTION('ref_axis',(1.,0.,0.));
#18445=DIRECTION('center_axis',(0.,1.,0.));
#18446=DIRECTION('ref_axis',(0.,0.,1.));
#18447=DIRECTION('',(-8.65956056235489E-17,0.70710678118655,-0.707106781186544));
#18448=DIRECTION('center_axis',(0.,1.,0.));
#18449=DIRECTION('ref_axis',(1.,0.,0.));
#18450=DIRECTION('center_axis',(0.,1.,0.));
#18451=DIRECTION('ref_axis',(0.707106781186549,0.,-0.707106781186546));
#18452=DIRECTION('center_axis',(0.,1.,0.));
#18453=DIRECTION('ref_axis',(-0.707106781186548,0.,-0.707106781186547));
#21059=CARTESIAN_POINT('',(0.,0.,0.));
#21060=CARTESIAN_POINT('Origin',(7.2,2.3,1.4));
#21061=CARTESIAN_POINT('',(7.2,2.3,1.4));
#21062=CARTESIAN_POINT('',(7.2,1.9,1.4));
#21063=CARTESIAN_POINT('',(7.2,1.15,1.4));
#21064=CARTESIAN_POINT('',(6.6,2.3,1.4));
#21065=CARTESIAN_POINT('',(7.2,2.3,1.4));
#21066=CARTESIAN_POINT('',(6.6,1.9,1.4));
#21067=CARTESIAN_POINT('',(6.6,1.9,1.4));
#21068=CARTESIAN_POINT('',(7.2,1.9,1.4));
#21069=CARTESIAN_POINT('Origin',(7.2,2.3,10.));
#21070=CARTESIAN_POINT('',(7.2,2.3,10.));
#21071=CARTESIAN_POINT('',(7.2,2.3,13.7));
#21072=CARTESIAN_POINT('',(6.6,2.3,10.));
#21073=CARTESIAN_POINT('',(7.2,2.3,10.));
#21074=CARTESIAN_POINT('',(6.6,2.3,1.4));
#21075=CARTESIAN_POINT('Origin',(7.2,1.9,10.));
#21076=CARTESIAN_POINT('',(7.2,1.9,10.));
#21077=CARTESIAN_POINT('',(7.2,0.95,10.));
#21078=CARTESIAN_POINT('',(6.6,1.9,10.));
#21079=CARTESIAN_POINT('',(7.2,1.9,10.));
#21080=CARTESIAN_POINT('',(6.6,2.3,10.));
#21081=CARTESIAN_POINT('Origin',(7.2,1.9,1.4));
#21082=CARTESIAN_POINT('',(7.2,1.9,9.4));
#21083=CARTESIAN_POINT('',(6.6,1.9,10.));
#21084=CARTESIAN_POINT('Origin',(6.6,2.1,5.7));
#21085=CARTESIAN_POINT('Origin',(7.2,-3.3,1.4));
#21086=CARTESIAN_POINT('',(7.2,-3.6,1.4));
#21087=CARTESIAN_POINT('',(6.6,-3.6,1.4));
#21088=CARTESIAN_POINT('',(6.625,-3.6,1.4));
#21089=CARTESIAN_POINT('',(7.2,-3.3,1.4));
#21090=CARTESIAN_POINT('',(7.2,-1.65,1.4));
#21091=CARTESIAN_POINT('',(6.6,-3.3,1.4));
#21092=CARTESIAN_POINT('',(7.2,-3.3,1.4));
#21093=CARTESIAN_POINT('',(6.6,-3.7,1.4));
#21094=CARTESIAN_POINT('Origin',(6.6,-3.5,5.7));
#21095=CARTESIAN_POINT('',(6.6,-3.6,3.4));
#21096=CARTESIAN_POINT('',(6.6,-3.6,4.));
#21097=CARTESIAN_POINT('',(6.6,-3.3,10.));
#21098=CARTESIAN_POINT('',(6.6,-3.3,1.4));
#21099=CARTESIAN_POINT('',(6.6,-3.7,10.));
#21100=CARTESIAN_POINT('',(6.6,-3.3,10.));
#21101=CARTESIAN_POINT('',(6.6,-3.7,3.4));
#21102=CARTESIAN_POINT('',(6.6,-3.7,10.));
#21103=CARTESIAN_POINT('',(6.6,-3.55,3.4));
#21104=CARTESIAN_POINT('Origin',(7.2,-3.3,10.));
#21105=CARTESIAN_POINT('',(7.2,-3.3,10.));
#21106=CARTESIAN_POINT('',(7.2,-3.3,13.7));
#21107=CARTESIAN_POINT('',(7.2,-3.3,10.));
#21108=CARTESIAN_POINT('Origin',(7.2,-3.7,10.));
#21109=CARTESIAN_POINT('',(7.2,-3.7,10.));
#21110=CARTESIAN_POINT('',(7.2,-1.85,10.));
#21111=CARTESIAN_POINT('',(7.2,-3.7,10.));
#21112=CARTESIAN_POINT('Origin',(7.2,-3.7,1.4));
#21113=CARTESIAN_POINT('',(7.2,-3.7,3.4));
#21114=CARTESIAN_POINT('',(7.25,-3.7,3.4));
#21115=CARTESIAN_POINT('',(7.2,-3.7,9.4));
#21116=CARTESIAN_POINT('Origin',(7.2,-1.9,1.4));
#21117=CARTESIAN_POINT('',(7.2,-1.9,1.4));
#21118=CARTESIAN_POINT('',(7.2,-2.3,1.4));
#21119=CARTESIAN_POINT('',(7.2,-0.95,1.4));
#21120=CARTESIAN_POINT('',(6.6,-1.9,1.4));
#21121=CARTESIAN_POINT('',(7.2,-1.9,1.4));
#21122=CARTESIAN_POINT('',(6.6,-2.3,1.4));
#21123=CARTESIAN_POINT('',(6.6,-2.3,1.4));
#21124=CARTESIAN_POINT('',(7.2,-2.3,1.4));
#21125=CARTESIAN_POINT('Origin',(7.2,-1.9,10.));
#21126=CARTESIAN_POINT('',(7.2,-1.9,10.));
#21127=CARTESIAN_POINT('',(7.2,-1.9,13.7));
#21128=CARTESIAN_POINT('',(6.6,-1.9,10.));
#21129=CARTESIAN_POINT('',(7.2,-1.9,10.));
#21130=CARTESIAN_POINT('',(6.6,-1.9,1.4));
#21131=CARTESIAN_POINT('Origin',(7.2,-2.3,10.));
#21132=CARTESIAN_POINT('',(7.2,-2.3,10.));
#21133=CARTESIAN_POINT('',(7.2,-1.15,10.));
#21134=CARTESIAN_POINT('',(6.6,-2.3,10.));
#21135=CARTESIAN_POINT('',(7.2,-2.3,10.));
#21136=CARTESIAN_POINT('',(6.6,-1.9,10.));
#21137=CARTESIAN_POINT('Origin',(7.2,-2.3,1.4));
#21138=CARTESIAN_POINT('',(7.2,-2.3,9.4));
#21139=CARTESIAN_POINT('',(6.6,-2.3,10.));
#21140=CARTESIAN_POINT('Origin',(6.6,-2.1,5.7));
#21141=CARTESIAN_POINT('Origin',(7.2,-0.5,1.4));
#21142=CARTESIAN_POINT('',(7.2,-0.5,1.4));
#21143=CARTESIAN_POINT('',(7.2,-0.9,1.4));
#21144=CARTESIAN_POINT('',(7.2,-0.25,1.4));
#21145=CARTESIAN_POINT('',(6.6,-0.5,1.4));
#21146=CARTESIAN_POINT('',(7.2,-0.5,1.4));
#21147=CARTESIAN_POINT('',(6.6,-0.9,1.4));
#21148=CARTESIAN_POINT('',(6.6,-0.9,1.4));
#21149=CARTESIAN_POINT('',(7.2,-0.9,1.4));
#21150=CARTESIAN_POINT('Origin',(7.2,-0.5,10.));
#21151=CARTESIAN_POINT('',(7.2,-0.5,10.));
#21152=CARTESIAN_POINT('',(7.2,-0.5,13.7));
#21153=CARTESIAN_POINT('',(6.6,-0.5,10.));
#21154=CARTESIAN_POINT('',(7.2,-0.5,10.));
#21155=CARTESIAN_POINT('',(6.6,-0.5,1.4));
#21156=CARTESIAN_POINT('Origin',(7.2,-0.9,10.));
#21157=CARTESIAN_POINT('',(7.2,-0.9,10.));
#21158=CARTESIAN_POINT('',(7.2,-0.45,10.));
#21159=CARTESIAN_POINT('',(6.6,-0.9,10.));
#21160=CARTESIAN_POINT('',(7.2,-0.9,10.));
#21161=CARTESIAN_POINT('',(6.6,-0.5,10.));
#21162=CARTESIAN_POINT('Origin',(7.2,-0.9,1.4));
#21163=CARTESIAN_POINT('',(7.2,-0.9,9.4));
#21164=CARTESIAN_POINT('',(6.6,-0.9,10.));
#21165=CARTESIAN_POINT('Origin',(6.6,-0.7,5.7));
#21166=CARTESIAN_POINT('Origin',(7.2,0.9,1.4));
#21167=CARTESIAN_POINT('',(7.2,0.9,1.4));
#21168=CARTESIAN_POINT('',(7.2,0.5,1.4));
#21169=CARTESIAN_POINT('',(7.2,0.45,1.4));
#21170=CARTESIAN_POINT('',(6.6,0.9,1.4));
#21171=CARTESIAN_POINT('',(7.2,0.9,1.4));
#21172=CARTESIAN_POINT('',(6.6,0.5,1.4));
#21173=CARTESIAN_POINT('',(6.6,0.5,1.4));
#21174=CARTESIAN_POINT('',(7.2,0.5,1.4));
#21175=CARTESIAN_POINT('Origin',(7.2,0.9,10.));
#21176=CARTESIAN_POINT('',(7.2,0.9,10.));
#21177=CARTESIAN_POINT('',(7.2,0.9,13.7));
#21178=CARTESIAN_POINT('',(6.6,0.9,10.));
#21179=CARTESIAN_POINT('',(7.2,0.9,10.));
#21180=CARTESIAN_POINT('',(6.6,0.9,1.4));
#21181=CARTESIAN_POINT('Origin',(7.2,0.5,10.));
#21182=CARTESIAN_POINT('',(7.2,0.5,10.));
#21183=CARTESIAN_POINT('',(7.2,0.25,10.));
#21184=CARTESIAN_POINT('',(6.6,0.5,10.));
#21185=CARTESIAN_POINT('',(7.2,0.5,10.));
#21186=CARTESIAN_POINT('',(6.6,0.9,10.));
#21187=CARTESIAN_POINT('Origin',(7.2,0.5,1.4));
#21188=CARTESIAN_POINT('',(7.2,0.5,9.4));
#21189=CARTESIAN_POINT('',(6.6,0.5,10.));
#21190=CARTESIAN_POINT('Origin',(6.6,0.7,5.7));
#21191=CARTESIAN_POINT('Origin',(7.2,3.7,1.4));
#21192=CARTESIAN_POINT('',(6.6,3.6,1.4));
#21193=CARTESIAN_POINT('',(7.2,3.6,1.4));
#21194=CARTESIAN_POINT('',(6.625,3.6,1.4));
#21195=CARTESIAN_POINT('',(6.6,3.3,1.4));
#21196=CARTESIAN_POINT('',(6.6,3.3,1.4));
#21197=CARTESIAN_POINT('',(7.2,3.3,1.4));
#21198=CARTESIAN_POINT('',(7.2,3.3,1.4));
#21199=CARTESIAN_POINT('',(7.2,1.85,1.4));
#21200=CARTESIAN_POINT('Origin',(7.2,3.7,10.));
#21201=CARTESIAN_POINT('',(7.2,3.7,3.4));
#21202=CARTESIAN_POINT('',(6.6,3.7,3.4));
#21203=CARTESIAN_POINT('',(6.,3.7,3.4));
#21204=CARTESIAN_POINT('',(7.2,3.7,10.));
#21205=CARTESIAN_POINT('',(7.2,3.7,13.7));
#21206=CARTESIAN_POINT('',(6.6,3.7,10.));
#21207=CARTESIAN_POINT('',(7.2,3.7,10.));
#21208=CARTESIAN_POINT('',(6.6,3.7,1.4));
#21209=CARTESIAN_POINT('Origin',(7.2,3.3,10.));
#21210=CARTESIAN_POINT('',(7.2,3.3,10.));
#21211=CARTESIAN_POINT('',(7.2,1.65,10.));
#21212=CARTESIAN_POINT('',(6.6,3.3,10.));
#21213=CARTESIAN_POINT('',(7.2,3.3,10.));
#21214=CARTESIAN_POINT('',(6.6,3.7,10.));
#21215=CARTESIAN_POINT('Origin',(7.2,3.3,1.4));
#21216=CARTESIAN_POINT('',(7.2,3.3,9.4));
#21217=CARTESIAN_POINT('',(6.6,3.3,10.));
#21218=CARTESIAN_POINT('Origin',(6.6,3.5,5.7));
#21219=CARTESIAN_POINT('',(6.6,3.6,3.4));
#21220=CARTESIAN_POINT('',(6.6,3.6,4.));
#21221=CARTESIAN_POINT('',(6.6,3.55,3.4));
#21222=CARTESIAN_POINT('Origin',(6.05,-3.6,2.3));
#21223=CARTESIAN_POINT('',(4.8,-3.6,3.4));
#21224=CARTESIAN_POINT('',(7.3,-3.6,3.4));
#21225=CARTESIAN_POINT('',(4.8,-3.6,1.2));
#21226=CARTESIAN_POINT('',(4.8,-3.6,3.4));
#21227=CARTESIAN_POINT('',(7.2,-3.6,1.2));
#21228=CARTESIAN_POINT('',(4.8,-3.6,1.2));
#21229=CARTESIAN_POINT('',(7.2,-3.6,9.85));
#21230=CARTESIAN_POINT('Origin',(7.3,-3.6,3.4));
#21231=CARTESIAN_POINT('',(7.2,-4.6,3.4));
#21232=CARTESIAN_POINT('',(7.2,-1.8,3.4));
#21233=CARTESIAN_POINT('',(4.8,-4.6,3.4));
#21234=CARTESIAN_POINT('',(3.65,-4.6,3.4));
#21235=CARTESIAN_POINT('',(4.8,-3.6,3.4));
#21236=CARTESIAN_POINT('Origin',(7.2,0.,17.4));
#21237=CARTESIAN_POINT('',(7.2,-4.6,1.2));
#21238=CARTESIAN_POINT('',(7.2,-1.8,1.2));
#21239=CARTESIAN_POINT('',(7.2,-4.6,0.6));
#21240=CARTESIAN_POINT('',(7.2,-4.6,0.));
#21241=CARTESIAN_POINT('',(7.2,4.6,0.6));
#21242=CARTESIAN_POINT('',(7.2,0.,0.6));
#21243=CARTESIAN_POINT('',(7.2,4.6,1.2));
#21244=CARTESIAN_POINT('',(7.2,4.6,0.));
#21245=CARTESIAN_POINT('',(7.2,3.6,1.2));
#21246=CARTESIAN_POINT('',(7.2,1.8,1.2));
#21247=CARTESIAN_POINT('',(7.2,3.6,9.85));
#21248=CARTESIAN_POINT('',(7.2,4.6,3.4));
#21249=CARTESIAN_POINT('',(7.2,1.8,3.4));
#21250=CARTESIAN_POINT('',(7.2,4.6,16.8));
#21251=CARTESIAN_POINT('',(7.2,4.6,0.));
#21252=CARTESIAN_POINT('',(7.2,-4.6,16.8));
#21253=CARTESIAN_POINT('',(7.2,0.,16.8));
#21254=CARTESIAN_POINT('',(7.2,-4.6,0.));
#21255=CARTESIAN_POINT('',(7.2,-3.18408167778312E-16,10.9));
#21256=CARTESIAN_POINT('Origin',(7.2,0.,13.5));
#21257=CARTESIAN_POINT('Origin',(-7.2,2.3,6.));
#21258=CARTESIAN_POINT('',(-7.2,2.3,6.));
#21259=CARTESIAN_POINT('',(-7.2,1.9,6.));
#21260=CARTESIAN_POINT('',(-7.2,1.15,6.));
#21261=CARTESIAN_POINT('',(-6.6,2.3,6.));
#21262=CARTESIAN_POINT('',(-7.2,2.3,6.));
#21263=CARTESIAN_POINT('',(-6.6,1.9,6.));
#21264=CARTESIAN_POINT('',(-6.6,2.3,6.));
#21265=CARTESIAN_POINT('',(-7.2,1.9,6.));
#21266=CARTESIAN_POINT('Origin',(-7.2,2.3,1.4));
#21267=CARTESIAN_POINT('',(-7.2,2.3,1.4));
#21268=CARTESIAN_POINT('',(-7.2,2.3,0.7));
#21269=CARTESIAN_POINT('',(-6.6,2.3,1.4));
#21270=CARTESIAN_POINT('',(-7.2,2.3,1.4));
#21271=CARTESIAN_POINT('',(-6.6,2.3,1.4));
#21272=CARTESIAN_POINT('Origin',(-7.2,1.9,1.4));
#21273=CARTESIAN_POINT('',(-7.2,1.9,1.4));
#21274=CARTESIAN_POINT('',(-7.2,0.95,1.4));
#21275=CARTESIAN_POINT('',(-6.6,1.9,1.4));
#21276=CARTESIAN_POINT('',(-7.2,1.9,1.4));
#21277=CARTESIAN_POINT('',(-6.6,1.9,1.4));
#21278=CARTESIAN_POINT('Origin',(-7.2,1.9,6.));
#21279=CARTESIAN_POINT('',(-7.2,1.9,3.));
#21280=CARTESIAN_POINT('',(-6.6,1.9,6.));
#21281=CARTESIAN_POINT('Origin',(-6.6,2.1,3.7));
#21282=CARTESIAN_POINT('Origin',(-7.2,-3.7,1.4));
#21283=CARTESIAN_POINT('',(-6.6,-3.6,1.4));
#21284=CARTESIAN_POINT('',(-7.2,-3.6,1.4));
#21285=CARTESIAN_POINT('',(-6.625,-3.6,1.4));
#21286=CARTESIAN_POINT('',(-6.6,-3.3,1.4));
#21287=CARTESIAN_POINT('',(-6.6,-3.7,1.4));
#21288=CARTESIAN_POINT('',(-7.2,-3.3,1.4));
#21289=CARTESIAN_POINT('',(-7.2,-3.3,1.4));
#21290=CARTESIAN_POINT('',(-7.2,-1.85,1.4));
#21291=CARTESIAN_POINT('Origin',(-7.2,-3.3,6.));
#21292=CARTESIAN_POINT('',(-7.2,-3.3,6.));
#21293=CARTESIAN_POINT('',(-7.2,-3.7,6.));
#21294=CARTESIAN_POINT('',(-7.2,-1.65,6.));
#21295=CARTESIAN_POINT('',(-6.6,-3.3,6.));
#21296=CARTESIAN_POINT('',(-7.2,-3.3,6.));
#21297=CARTESIAN_POINT('',(-6.6,-3.7,6.));
#21298=CARTESIAN_POINT('',(-6.6,-3.3,6.));
#21299=CARTESIAN_POINT('',(-7.2,-3.7,6.));
#21300=CARTESIAN_POINT('Origin',(-7.2,-3.3,1.4));
#21301=CARTESIAN_POINT('',(-7.2,-3.3,0.7));
#21302=CARTESIAN_POINT('',(-6.6,-3.3,1.4));
#21303=CARTESIAN_POINT('Origin',(-7.2,-3.7,6.));
#21304=CARTESIAN_POINT('',(-7.2,-3.7,3.4));
#21305=CARTESIAN_POINT('',(-6.6,-3.7,3.4));
#21306=CARTESIAN_POINT('',(-6.,-3.7,3.4));
#21307=CARTESIAN_POINT('',(-7.2,-3.7,3.));
#21308=CARTESIAN_POINT('',(-6.6,-3.7,6.));
#21309=CARTESIAN_POINT('Origin',(-6.6,-3.5,3.7));
#21310=CARTESIAN_POINT('',(-6.6,-3.6,3.4));
#21311=CARTESIAN_POINT('',(-6.6,-3.6,3.));
#21312=CARTESIAN_POINT('',(-6.6,-3.55,3.4));
#21313=CARTESIAN_POINT('Origin',(-7.2,-1.9,6.));
#21314=CARTESIAN_POINT('',(-7.2,-1.9,6.));
#21315=CARTESIAN_POINT('',(-7.2,-2.3,6.));
#21316=CARTESIAN_POINT('',(-7.2,-0.95,6.));
#21317=CARTESIAN_POINT('',(-6.6,-1.9,6.));
#21318=CARTESIAN_POINT('',(-7.2,-1.9,6.));
#21319=CARTESIAN_POINT('',(-6.6,-2.3,6.));
#21320=CARTESIAN_POINT('',(-6.6,-1.9,6.));
#21321=CARTESIAN_POINT('',(-7.2,-2.3,6.));
#21322=CARTESIAN_POINT('Origin',(-7.2,-1.9,1.4));
#21323=CARTESIAN_POINT('',(-7.2,-1.9,1.4));
#21324=CARTESIAN_POINT('',(-7.2,-1.9,0.7));
#21325=CARTESIAN_POINT('',(-6.6,-1.9,1.4));
#21326=CARTESIAN_POINT('',(-7.2,-1.9,1.4));
#21327=CARTESIAN_POINT('',(-6.6,-1.9,1.4));
#21328=CARTESIAN_POINT('Origin',(-7.2,-2.3,1.4));
#21329=CARTESIAN_POINT('',(-7.2,-2.3,1.4));
#21330=CARTESIAN_POINT('',(-7.2,-1.15,1.4));
#21331=CARTESIAN_POINT('',(-6.6,-2.3,1.4));
#21332=CARTESIAN_POINT('',(-7.2,-2.3,1.4));
#21333=CARTESIAN_POINT('',(-6.6,-2.3,1.4));
#21334=CARTESIAN_POINT('Origin',(-7.2,-2.3,6.));
#21335=CARTESIAN_POINT('',(-7.2,-2.3,3.));
#21336=CARTESIAN_POINT('',(-6.6,-2.3,6.));
#21337=CARTESIAN_POINT('Origin',(-6.6,-2.1,3.7));
#21338=CARTESIAN_POINT('Origin',(-7.2,-0.5,6.));
#21339=CARTESIAN_POINT('',(-7.2,-0.5,6.));
#21340=CARTESIAN_POINT('',(-7.2,-0.9,6.));
#21341=CARTESIAN_POINT('',(-7.2,-0.25,6.));
#21342=CARTESIAN_POINT('',(-6.6,-0.5,6.));
#21343=CARTESIAN_POINT('',(-7.2,-0.5,6.));
#21344=CARTESIAN_POINT('',(-6.6,-0.9,6.));
#21345=CARTESIAN_POINT('',(-6.6,-0.5,6.));
#21346=CARTESIAN_POINT('',(-7.2,-0.9,6.));
#21347=CARTESIAN_POINT('Origin',(-7.2,-0.5,1.4));
#21348=CARTESIAN_POINT('',(-7.2,-0.5,1.4));
#21349=CARTESIAN_POINT('',(-7.2,-0.5,0.7));
#21350=CARTESIAN_POINT('',(-6.6,-0.5,1.4));
#21351=CARTESIAN_POINT('',(-7.2,-0.5,1.4));
#21352=CARTESIAN_POINT('',(-6.6,-0.5,1.4));
#21353=CARTESIAN_POINT('Origin',(-7.2,-0.9,1.4));
#21354=CARTESIAN_POINT('',(-7.2,-0.9,1.4));
#21355=CARTESIAN_POINT('',(-7.2,-0.45,1.4));
#21356=CARTESIAN_POINT('',(-6.6,-0.9,1.4));
#21357=CARTESIAN_POINT('',(-7.2,-0.9,1.4));
#21358=CARTESIAN_POINT('',(-6.6,-0.9,1.4));
#21359=CARTESIAN_POINT('Origin',(-7.2,-0.9,6.));
#21360=CARTESIAN_POINT('',(-7.2,-0.9,3.));
#21361=CARTESIAN_POINT('',(-6.6,-0.9,6.));
#21362=CARTESIAN_POINT('Origin',(-6.6,-0.7,3.7));
#21363=CARTESIAN_POINT('Origin',(-7.2,0.9,6.));
#21364=CARTESIAN_POINT('',(-7.2,0.9,6.));
#21365=CARTESIAN_POINT('',(-7.2,0.5,6.));
#21366=CARTESIAN_POINT('',(-7.2,0.45,6.));
#21367=CARTESIAN_POINT('',(-6.6,0.9,6.));
#21368=CARTESIAN_POINT('',(-7.2,0.9,6.));
#21369=CARTESIAN_POINT('',(-6.6,0.5,6.));
#21370=CARTESIAN_POINT('',(-6.6,0.9,6.));
#21371=CARTESIAN_POINT('',(-7.2,0.5,6.));
#21372=CARTESIAN_POINT('Origin',(-7.2,0.9,1.4));
#21373=CARTESIAN_POINT('',(-7.2,0.9,1.4));
#21374=CARTESIAN_POINT('',(-7.2,0.9,0.7));
#21375=CARTESIAN_POINT('',(-6.6,0.9,1.4));
#21376=CARTESIAN_POINT('',(-7.2,0.9,1.4));
#21377=CARTESIAN_POINT('',(-6.6,0.9,1.4));
#21378=CARTESIAN_POINT('Origin',(-7.2,0.5,1.4));
#21379=CARTESIAN_POINT('',(-7.2,0.5,1.4));
#21380=CARTESIAN_POINT('',(-7.2,0.25,1.4));
#21381=CARTESIAN_POINT('',(-6.6,0.5,1.4));
#21382=CARTESIAN_POINT('',(-7.2,0.5,1.4));
#21383=CARTESIAN_POINT('',(-6.6,0.5,1.4));
#21384=CARTESIAN_POINT('Origin',(-7.2,0.5,6.));
#21385=CARTESIAN_POINT('',(-7.2,0.5,3.));
#21386=CARTESIAN_POINT('',(-6.6,0.5,6.));
#21387=CARTESIAN_POINT('Origin',(-6.6,0.7,3.7));
#21388=CARTESIAN_POINT('Origin',(-7.2,3.7,1.4));
#21389=CARTESIAN_POINT('',(-6.6,3.7,3.4));
#21390=CARTESIAN_POINT('',(-7.2,3.7,3.4));
#21391=CARTESIAN_POINT('',(-7.25,3.7,3.4));
#21392=CARTESIAN_POINT('',(-6.6,3.7,6.));
#21393=CARTESIAN_POINT('',(-6.6,3.7,1.4));
#21394=CARTESIAN_POINT('',(-7.2,3.7,6.));
#21395=CARTESIAN_POINT('',(-7.2,3.7,6.));
#21396=CARTESIAN_POINT('',(-7.2,3.7,0.7));
#21397=CARTESIAN_POINT('Origin',(-7.2,3.7,6.));
#21398=CARTESIAN_POINT('',(-7.2,3.3,6.));
#21399=CARTESIAN_POINT('',(-7.2,1.85,6.));
#21400=CARTESIAN_POINT('',(-6.6,3.3,6.));
#21401=CARTESIAN_POINT('',(-6.6,3.7,6.));
#21402=CARTESIAN_POINT('',(-7.2,3.3,6.));
#21403=CARTESIAN_POINT('Origin',(-7.2,3.3,1.4));
#21404=CARTESIAN_POINT('',(-7.2,3.6,1.4));
#21405=CARTESIAN_POINT('',(-6.6,3.6,1.4));
#21406=CARTESIAN_POINT('',(-6.625,3.6,1.4));
#21407=CARTESIAN_POINT('',(-7.2,3.3,1.4));
#21408=CARTESIAN_POINT('',(-7.2,1.65,1.4));
#21409=CARTESIAN_POINT('',(-6.6,3.3,1.4));
#21410=CARTESIAN_POINT('',(-7.2,3.3,1.4));
#21411=CARTESIAN_POINT('',(-6.6,3.3,1.4));
#21412=CARTESIAN_POINT('Origin',(-7.2,3.3,6.));
#21413=CARTESIAN_POINT('',(-7.2,3.3,3.));
#21414=CARTESIAN_POINT('',(-6.6,3.3,6.));
#21415=CARTESIAN_POINT('Origin',(-6.6,3.5,3.7));
#21416=CARTESIAN_POINT('',(-6.6,3.6,3.4));
#21417=CARTESIAN_POINT('',(-6.6,3.55,3.4));
#21418=CARTESIAN_POINT('',(-6.6,3.6,3.));
#21419=CARTESIAN_POINT('Origin',(-6.05,-3.6,2.3));
#21420=CARTESIAN_POINT('',(-7.2,-3.6,1.2));
#21421=CARTESIAN_POINT('',(-7.2,-3.6,1.15));
#21422=CARTESIAN_POINT('',(-4.8,-3.6,1.2));
#21423=CARTESIAN_POINT('',(-7.3,-3.6,1.2));
#21424=CARTESIAN_POINT('',(-4.8,-3.6,3.4));
#21425=CARTESIAN_POINT('',(-4.8,-3.6,1.2));
#21426=CARTESIAN_POINT('',(-4.8,-3.6,3.4));
#21427=CARTESIAN_POINT('Origin',(-7.3,3.6,3.4));
#21428=CARTESIAN_POINT('',(-7.2,4.6,3.4));
#21429=CARTESIAN_POINT('',(-7.2,1.8,3.4));
#21430=CARTESIAN_POINT('',(-4.8,4.6,3.4));
#21431=CARTESIAN_POINT('',(-3.65,4.6,3.4));
#21432=CARTESIAN_POINT('',(-4.8,3.6,3.4));
#21433=CARTESIAN_POINT('',(-4.8,3.6,3.4));
#21434=CARTESIAN_POINT('',(-4.8,3.6,3.4));
#21435=CARTESIAN_POINT('Origin',(-7.2,0.,0.));
#21436=CARTESIAN_POINT('',(-7.2,-4.6,3.4));
#21437=CARTESIAN_POINT('',(-7.2,-1.8,3.4));
#21438=CARTESIAN_POINT('',(-7.2,-4.6,16.8));
#21439=CARTESIAN_POINT('',(-7.2,-4.6,17.4));
#21440=CARTESIAN_POINT('',(-7.2,-3.51681487422156,16.8));
#21441=CARTESIAN_POINT('',(-7.2,0.,16.8));
#21442=CARTESIAN_POINT('',(-7.2,-2.827,16.682));
#21443=CARTESIAN_POINT('Origin',(-7.2,-3.182,16.682));
#21444=CARTESIAN_POINT('',(-7.2,-2.84718512577844,16.8));
#21445=CARTESIAN_POINT('Origin',(-7.2,-3.182,16.682));
#21446=CARTESIAN_POINT('',(-7.2,2.84718512577844,16.8));
#21447=CARTESIAN_POINT('',(-7.2,0.,16.8));
#21448=CARTESIAN_POINT('',(-7.2,3.537,16.682));
#21449=CARTESIAN_POINT('Origin',(-7.2,3.182,16.682));
#21450=CARTESIAN_POINT('',(-7.2,3.51681487422156,16.8));
#21451=CARTESIAN_POINT('Origin',(-7.2,3.182,16.682));
#21452=CARTESIAN_POINT('',(-7.2,4.6,16.8));
#21453=CARTESIAN_POINT('',(-7.2,0.,16.8));
#21454=CARTESIAN_POINT('',(-7.2,4.6,17.4));
#21455=CARTESIAN_POINT('',(-7.2,3.6,1.2));
#21456=CARTESIAN_POINT('',(-7.2,3.6,1.15));
#21457=CARTESIAN_POINT('',(-7.2,4.6,1.2));
#21458=CARTESIAN_POINT('',(-7.2,1.8,1.2));
#21459=CARTESIAN_POINT('',(-7.2,4.6,0.600000000000001));
#21460=CARTESIAN_POINT('',(-7.2,4.6,17.4));
#21461=CARTESIAN_POINT('',(-7.2,-4.6,0.600000000000001));
#21462=CARTESIAN_POINT('',(-7.2,0.,0.6));
#21463=CARTESIAN_POINT('',(-7.2,-4.6,1.2));
#21464=CARTESIAN_POINT('',(-7.2,-4.6,17.4));
#21465=CARTESIAN_POINT('',(-7.2,-1.8,1.2));
#21466=CARTESIAN_POINT('',(-7.2,-3.18408167778312E-16,10.9));
#21467=CARTESIAN_POINT('Origin',(-7.2,0.,13.5));
#21468=CARTESIAN_POINT('',(-7.2,3.537,10.318));
#21469=CARTESIAN_POINT('Origin',(-7.2,3.182,10.318));
#21470=CARTESIAN_POINT('',(-7.2,-2.827,10.318));
#21471=CARTESIAN_POINT('Origin',(-7.2,-3.182,10.318));
#21472=CARTESIAN_POINT('Origin',(0.,-4.6,7.2));
#21473=CARTESIAN_POINT('',(5.57660788571496,-4.6,8.79419085713778));
#21474=CARTESIAN_POINT('',(-5.57660788571496,-4.6,8.79419085713778));
#21475=CARTESIAN_POINT('Origin',(0.,-4.6,7.2));
#21476=CARTESIAN_POINT('',(5.57660788571496,-4.1,8.79419085713778));
#21477=CARTESIAN_POINT('',(5.57660788571496,-4.6,8.79419085713778));
#21478=CARTESIAN_POINT('',(-5.57660788571496,-4.1,8.79419085713778));
#21479=CARTESIAN_POINT('Origin',(0.,-4.1,7.2));
#21480=CARTESIAN_POINT('',(-5.57660788571496,-4.6,8.79419085713778));
#21481=CARTESIAN_POINT('Origin',(6.,-4.6,8.));
#21482=CARTESIAN_POINT('',(6.4,-4.6,8.80622577482985));
#21483=CARTESIAN_POINT('Origin',(6.,-4.6,8.));
#21484=CARTESIAN_POINT('',(6.4,-4.1,8.80622577482985));
#21485=CARTESIAN_POINT('',(6.4,-4.6,8.80622577482985));
#21486=CARTESIAN_POINT('Origin',(6.,-4.1,8.));
#21487=CARTESIAN_POINT('Origin',(6.4,-4.6,16.));
#21488=CARTESIAN_POINT('',(6.4,-4.6,16.));
#21489=CARTESIAN_POINT('',(6.4,-4.6,12.35));
#21490=CARTESIAN_POINT('',(6.4,-4.1,16.));
#21491=CARTESIAN_POINT('',(6.4,-4.6,16.));
#21492=CARTESIAN_POINT('',(6.4,-4.1,1.4));
#21493=CARTESIAN_POINT('Origin',(-6.4,-4.6,16.));
#21494=CARTESIAN_POINT('',(-6.4,-4.6,16.));
#21495=CARTESIAN_POINT('',(-3.2,-4.6,16.));
#21496=CARTESIAN_POINT('',(-6.4,-4.1,16.));
#21497=CARTESIAN_POINT('',(-6.4,-4.6,16.));
#21498=CARTESIAN_POINT('',(6.4,-4.1,16.));
#21499=CARTESIAN_POINT('Origin',(-6.4,-4.6,8.80622577482985));
#21500=CARTESIAN_POINT('',(-6.4,-4.6,8.80622577482985));
#21501=CARTESIAN_POINT('',(-6.4,-4.6,8.75311288741493));
#21502=CARTESIAN_POINT('',(-6.4,-4.1,8.80622577482985));
#21503=CARTESIAN_POINT('',(-6.4,-4.6,8.80622577482985));
#21504=CARTESIAN_POINT('',(-6.4,-4.1,16.));
#21505=CARTESIAN_POINT('Origin',(-6.,-4.6,8.));
#21506=CARTESIAN_POINT('Origin',(-6.,-4.6,8.));
#21507=CARTESIAN_POINT('Origin',(-6.,-4.1,8.));
#21508=CARTESIAN_POINT('Origin',(0.,-4.1,12.3970954285689));
#21509=CARTESIAN_POINT('Origin',(-6.4,4.6,16.));
#21510=CARTESIAN_POINT('',(-6.4,4.6,16.));
#21511=CARTESIAN_POINT('',(-6.4,4.6,8.80622577482985));
#21512=CARTESIAN_POINT('',(-6.4,4.6,12.35));
#21513=CARTESIAN_POINT('',(-6.4,4.1,16.));
#21514=CARTESIAN_POINT('',(-6.4,4.6,16.));
#21515=CARTESIAN_POINT('',(-6.4,4.1,8.80622577482985));
#21516=CARTESIAN_POINT('',(-6.4,4.1,16.));
#21517=CARTESIAN_POINT('',(-6.4,4.6,8.80622577482985));
#21518=CARTESIAN_POINT('Origin',(6.4,4.6,16.));
#21519=CARTESIAN_POINT('',(6.4,4.6,16.));
#21520=CARTESIAN_POINT('',(3.2,4.6,16.));
#21521=CARTESIAN_POINT('',(6.4,4.1,16.));
#21522=CARTESIAN_POINT('',(6.4,4.6,16.));
#21523=CARTESIAN_POINT('',(6.4,4.1,16.));
#21524=CARTESIAN_POINT('Origin',(6.4,4.6,8.80622577482985));
#21525=CARTESIAN_POINT('',(6.4,4.6,8.80622577482985));
#21526=CARTESIAN_POINT('',(6.4,4.6,8.75311288741493));
#21527=CARTESIAN_POINT('',(6.4,4.1,8.80622577482985));
#21528=CARTESIAN_POINT('',(6.4,4.6,8.80622577482985));
#21529=CARTESIAN_POINT('',(6.4,4.1,1.4));
#21530=CARTESIAN_POINT('Origin',(0.,4.1,12.3970954285689));
#21531=CARTESIAN_POINT('',(-5.57660788571496,4.1,8.79419085713778));
#21532=CARTESIAN_POINT('Origin',(-6.,4.1,8.));
#21533=CARTESIAN_POINT('',(5.57660788571496,4.1,8.79419085713778));
#21534=CARTESIAN_POINT('Origin',(6.,4.1,8.));
#21535=CARTESIAN_POINT('Origin',(0.,4.1,7.2));
#21536=CARTESIAN_POINT('Origin',(0.,4.6,8.7));
#21537=CARTESIAN_POINT('',(-5.79948381734181,4.6,7.12262136993645));
#21538=CARTESIAN_POINT('Origin',(-6.,4.6,8.));
#21539=CARTESIAN_POINT('',(-4.39098268679659,4.6,3.41063711895356));
#21540=CARTESIAN_POINT('Origin',(0.,4.6,7.2));
#21541=CARTESIAN_POINT('',(-4.8,4.6,3.01231056256177));
#21542=CARTESIAN_POINT('Origin',(-4.,4.6,2.6));
#21543=CARTESIAN_POINT('',(-4.8,4.6,6.05));
#21544=CARTESIAN_POINT('',(-6.6,4.6,17.4));
#21545=CARTESIAN_POINT('Origin',(-6.6,4.6,16.8));
#21546=CARTESIAN_POINT('',(6.6,4.6,17.4));
#21547=CARTESIAN_POINT('',(7.2,4.6,17.4));
#21548=CARTESIAN_POINT('Origin',(6.6,4.6,16.8));
#21549=CARTESIAN_POINT('',(4.8,4.6,3.4));
#21550=CARTESIAN_POINT('',(2.4,4.6,3.4));
#21551=CARTESIAN_POINT('',(4.8,4.6,3.01231056256177));
#21552=CARTESIAN_POINT('',(4.8,4.6,4.95));
#21553=CARTESIAN_POINT('',(4.39098268679659,4.6,3.41063711895356));
#21554=CARTESIAN_POINT('Origin',(4.,4.6,2.6));
#21555=CARTESIAN_POINT('',(5.79948381734181,4.6,7.12262136993645));
#21556=CARTESIAN_POINT('Origin',(0.,4.6,7.2));
#21557=CARTESIAN_POINT('Origin',(6.,4.6,8.));
#21558=CARTESIAN_POINT('Origin',(0.,5.55,7.2));
#21559=CARTESIAN_POINT('',(-5.69969977760644,5.6,7.25850166795172));
#21560=CARTESIAN_POINT('',(-4.22058574132406,5.6,3.36898760115136));
#21561=CARTESIAN_POINT('Origin',(0.,5.6,7.2));
#21562=CARTESIAN_POINT('',(-4.39098268679659,5.5,3.41063711895356));
#21563=CARTESIAN_POINT('Ctrl Pts',(-4.22058574132406,5.6,3.36898760115136));
#21564=CARTESIAN_POINT('Ctrl Pts',(-4.27772143963443,5.56861968092285,3.38524395544776));
#21565=CARTESIAN_POINT('Ctrl Pts',(-4.33480274427802,5.53491157572285,3.39897341264218));
#21566=CARTESIAN_POINT('Ctrl Pts',(-4.39098268679659,5.5,3.41063711895356));
#21567=CARTESIAN_POINT('',(-5.79948381734181,5.5,7.12262136993645));
#21568=CARTESIAN_POINT('Origin',(0.,5.5,7.2));
#21569=CARTESIAN_POINT('Ctrl Pts',(-5.69969977760644,5.6,7.25850166795172));
#21570=CARTESIAN_POINT('Ctrl Pts',(-5.73181372922814,5.56837145414589,7.21137187414533));
#21571=CARTESIAN_POINT('Ctrl Pts',(-5.76536271654192,5.53469693041621,7.16601092713632));
#21572=CARTESIAN_POINT('Ctrl Pts',(-5.79948381734181,5.5,7.12262136993645));
#21573=CARTESIAN_POINT('Origin',(-4.,5.55,2.6));
#21574=CARTESIAN_POINT('',(-4.7,5.6,2.98729833462074));
#21575=CARTESIAN_POINT('Origin',(-4.,5.6,2.6));
#21576=CARTESIAN_POINT('',(-4.8,5.5,3.01231056256177));
#21577=CARTESIAN_POINT('Origin',(-110.862782237101,-100.562782237101,2.99768857927433));
#21578=CARTESIAN_POINT('Origin',(-4.,5.5,2.6));
#21579=CARTESIAN_POINT('Origin',(-4.75,5.55,5.3));
#21580=CARTESIAN_POINT('',(-4.7,5.6,2.21270166537926));
#21581=CARTESIAN_POINT('',(-4.7,5.6,5.3));
#21582=CARTESIAN_POINT('',(-4.8,5.5,2.18768943743823));
#21583=CARTESIAN_POINT('Origin',(-110.862909719179,-100.562909719179,2.20231142463878));
#21584=CARTESIAN_POINT('',(-4.8,5.5,5.3));
#21585=CARTESIAN_POINT('Origin',(-4.,5.55,2.6));
#21586=CARTESIAN_POINT('',(-3.20783191206668,5.6,2.48833209744929));
#21587=CARTESIAN_POINT('Origin',(-4.,5.6,2.6));
#21588=CARTESIAN_POINT('',(-3.14292474054464,5.5,2.32536933960403));
#21589=CARTESIAN_POINT('Ctrl Pts',(-3.20783191206668,5.6,2.48833209744929));
#21590=CARTESIAN_POINT('Ctrl Pts',(-3.18379924141574,5.56861968092285,2.43400726134455));
#21591=CARTESIAN_POINT('Ctrl Pts',(-3.16227654075062,5.53491157572284,2.37938540957487));
#21592=CARTESIAN_POINT('Ctrl Pts',(-3.14292474054464,5.5,2.32536933960403));
#21593=CARTESIAN_POINT('Origin',(-4.,5.5,2.6));
#21594=CARTESIAN_POINT('Origin',(0.,5.55,7.2));
#21595=CARTESIAN_POINT('',(3.20783191206668,5.6,2.48833209744929));
#21596=CARTESIAN_POINT('Origin',(0.,5.6,7.2));
#21597=CARTESIAN_POINT('',(3.14292474054464,5.5,2.32536933960403));
#21598=CARTESIAN_POINT('Ctrl Pts',(3.20783191206668,5.6,2.48833209744929));
#21599=CARTESIAN_POINT('Ctrl Pts',(3.18379924141574,5.56861968092285,2.43400726134454));
#21600=CARTESIAN_POINT('Ctrl Pts',(3.16227654075062,5.53491157572284,2.37938540957487));
#21601=CARTESIAN_POINT('Ctrl Pts',(3.14292474054464,5.5,2.32536933960403));
#21602=CARTESIAN_POINT('Origin',(0.,5.5,7.2));
#21603=CARTESIAN_POINT('Origin',(4.,5.55,2.6));
#21604=CARTESIAN_POINT('',(4.7,5.6,2.21270166537926));
#21605=CARTESIAN_POINT('Origin',(4.,5.6,2.6));
#21606=CARTESIAN_POINT('',(4.8,5.5,2.18768943743823));
#21607=CARTESIAN_POINT('Origin',(110.863125461215,-100.563125461335,2.20231141751144));
#21608=CARTESIAN_POINT('Origin',(4.,5.5,2.6));
#21609=CARTESIAN_POINT('Origin',(4.75,5.55,4.2));
#21610=CARTESIAN_POINT('',(4.7,5.6,2.98729833462074));
#21611=CARTESIAN_POINT('',(4.7,5.6,4.2));
#21612=CARTESIAN_POINT('',(4.8,5.5,3.01231056256177));
#21613=CARTESIAN_POINT('Origin',(110.863314523851,-100.563314523971,2.99768857098632));
#21614=CARTESIAN_POINT('',(4.8,5.5,4.2));
#21615=CARTESIAN_POINT('Origin',(4.,5.55,2.6));
#21616=CARTESIAN_POINT('',(4.39098268679659,5.5,3.41063711895356));
#21617=CARTESIAN_POINT('Origin',(4.,5.5,2.6));
#21618=CARTESIAN_POINT('',(4.22058574132406,5.6,3.36898760115135));
#21619=CARTESIAN_POINT('Origin',(4.,5.6,2.6));
#21620=CARTESIAN_POINT('Ctrl Pts',(4.22058574132406,5.6,3.36898760115136));
#21621=CARTESIAN_POINT('Ctrl Pts',(4.27772143963443,5.56861968092285,3.38524395544776));
#21622=CARTESIAN_POINT('Ctrl Pts',(4.33480274427803,5.53491157572284,3.39897341264218));
#21623=CARTESIAN_POINT('Ctrl Pts',(4.39098268679659,5.5,3.41063711895356));
#21624=CARTESIAN_POINT('Origin',(0.,5.55,7.2));
#21625=CARTESIAN_POINT('',(5.79948381734181,5.5,7.12262136993645));
#21626=CARTESIAN_POINT('Origin',(0.,5.5,7.2));
#21627=CARTESIAN_POINT('',(5.69969977760644,5.6,7.25850166795172));
#21628=CARTESIAN_POINT('Origin',(0.,5.6,7.2));
#21629=CARTESIAN_POINT('Ctrl Pts',(5.69969977760644,5.6,7.25850166795172));
#21630=CARTESIAN_POINT('Ctrl Pts',(5.73181372922814,5.56837145414589,7.21137187414533));
#21631=CARTESIAN_POINT('Ctrl Pts',(5.76536271654191,5.53469693041622,7.16601092713632));
#21632=CARTESIAN_POINT('Ctrl Pts',(5.79948381734181,5.5,7.12262136993645));
#21633=CARTESIAN_POINT('Origin',(6.,5.55,8.));
#21634=CARTESIAN_POINT('',(5.57660788571496,5.5,8.79419085713778));
#21635=CARTESIAN_POINT('Origin',(6.,5.5,8.));
#21636=CARTESIAN_POINT('',(5.51591157610535,5.6,8.63691317920985));
#21637=CARTESIAN_POINT('Origin',(6.,5.6,8.));
#21638=CARTESIAN_POINT('Ctrl Pts',(5.51591157610535,5.6,8.63691317920985));
#21639=CARTESIAN_POINT('Ctrl Pts',(5.53455522536305,5.56837145414589,8.6908106531335));
#21640=CARTESIAN_POINT('Ctrl Pts',(5.55504723137093,5.53469693041621,8.74337706591873));
#21641=CARTESIAN_POINT('Ctrl Pts',(5.57660788571496,5.5,8.79419085713778));
#21642=CARTESIAN_POINT('Origin',(0.,5.55,7.2));
#21643=CARTESIAN_POINT('',(-5.57660788571496,5.5,8.79419085713778));
#21644=CARTESIAN_POINT('Origin',(0.,5.5,7.2));
#21645=CARTESIAN_POINT('',(-5.51591157610535,5.6,8.63691317920985));
#21646=CARTESIAN_POINT('Origin',(0.,5.6,7.2));
#21647=CARTESIAN_POINT('Ctrl Pts',(-5.51591157610535,5.6,8.63691317920985));
#21648=CARTESIAN_POINT('Ctrl Pts',(-5.53455522536306,5.56837145414589,8.6908106531335));
#21649=CARTESIAN_POINT('Ctrl Pts',(-5.55504723137093,5.53469693041621,8.74337706591873));
#21650=CARTESIAN_POINT('Ctrl Pts',(-5.57660788571496,5.5,8.79419085713779));
#21651=CARTESIAN_POINT('Origin',(-6.,5.55,8.));
#21652=CARTESIAN_POINT('Origin',(-6.,5.5,8.));
#21653=CARTESIAN_POINT('Origin',(-6.,5.6,8.));
#21654=CARTESIAN_POINT('Origin',(4.,4.6,2.6));
#21655=CARTESIAN_POINT('',(4.39098268679659,4.6,3.41063711895356));
#21656=CARTESIAN_POINT('',(4.8,4.6,3.01231056256177));
#21657=CARTESIAN_POINT('Origin',(0.,4.6,7.2));
#21658=CARTESIAN_POINT('',(5.79948381734181,4.6,7.12262136993645));
#21659=CARTESIAN_POINT('Origin',(6.,4.6,8.));
#21660=CARTESIAN_POINT('',(5.57660788571496,4.6,8.79419085713778));
#21661=CARTESIAN_POINT('Origin',(0.,4.6,7.2));
#21662=CARTESIAN_POINT('',(-5.57660788571496,4.6,8.79419085713778));
#21663=CARTESIAN_POINT('Origin',(-6.,4.6,8.));
#21664=CARTESIAN_POINT('',(-5.79948381734181,4.6,7.12262136993645));
#21665=CARTESIAN_POINT('Origin',(0.,4.6,7.2));
#21666=CARTESIAN_POINT('',(-4.39098268679659,4.6,3.41063711895356));
#21667=CARTESIAN_POINT('Origin',(0.,5.6,7.2));
#21668=CARTESIAN_POINT('',(3.85763741731416E-16,5.6,4.05));
#21669=CARTESIAN_POINT('Origin',(0.,5.6,7.2));
#21670=CARTESIAN_POINT('',(6.355,5.6,8.));
#21671=CARTESIAN_POINT('Origin',(6.,5.6,8.));
#21672=CARTESIAN_POINT('',(-5.645,5.6,8.));
#21673=CARTESIAN_POINT('Origin',(-6.,5.6,8.));
#21674=CARTESIAN_POINT('',(4.355,5.6,2.6));
#21675=CARTESIAN_POINT('Origin',(4.,5.6,2.6));
#21676=CARTESIAN_POINT('',(-3.645,5.6,2.6));
#21677=CARTESIAN_POINT('Origin',(-4.,5.6,2.6));
#21678=CARTESIAN_POINT('Origin',(-2.,0.,16.4725));
#21679=CARTESIAN_POINT('',(-2.,0.505,15.7438749965183));
#21680=CARTESIAN_POINT('',(-2.505,-2.39834377745635E-17,15.8));
#21681=CARTESIAN_POINT('Ctrl Pts',(-2.,0.505,15.7438749965183));
#21682=CARTESIAN_POINT('Ctrl Pts',(-2.06363520780063,0.505,15.7438749965183));
#21683=CARTESIAN_POINT('Ctrl Pts',(-2.13136458034946,0.492239912224197,
15.7468631623588));
#21684=CARTESIAN_POINT('Ctrl Pts',(-2.25572131394491,0.440639774787125,
15.7575497283031));
#21685=CARTESIAN_POINT('Ctrl Pts',(-2.31236734386936,0.401810505129054,
15.7650822805951));
#21686=CARTESIAN_POINT('Ctrl Pts',(-2.40180683616854,0.312371012829873,
15.7791387482964));
#21687=CARTESIAN_POINT('Ctrl Pts',(-2.44063897524859,0.255723435800378,
15.7865912587439));
#21688=CARTESIAN_POINT('Ctrl Pts',(-2.49224119847989,0.131361285500179,
15.7970934401131));
#21689=CARTESIAN_POINT('Ctrl Pts',(-2.505,0.0636299871652783,15.8));
#21690=CARTESIAN_POINT('Ctrl Pts',(-2.505,6.93889390390723E-17,15.8));
#21691=CARTESIAN_POINT('Ctrl Pts',(-2.505,6.93889390390723E-17,15.8));
#21692=CARTESIAN_POINT('Ctrl Pts',(-2.505,-0.0636299871652782,15.8));
#21693=CARTESIAN_POINT('Ctrl Pts',(-2.49224119847989,-0.131361285500179,
15.7970934401131));
#21694=CARTESIAN_POINT('Ctrl Pts',(-2.44063897524859,-0.255723435800378,
15.7865912587439));
#21695=CARTESIAN_POINT('Ctrl Pts',(-2.40180683616854,-0.312371012829873,
15.7791387482964));
#21696=CARTESIAN_POINT('Ctrl Pts',(-2.31236734386936,-0.401810505129054,
15.7650822805951));
#21697=CARTESIAN_POINT('Ctrl Pts',(-2.25572131394491,-0.440639774787125,
15.7575497283031));
#21698=CARTESIAN_POINT('Ctrl Pts',(-2.13136458034946,-0.492239912224197,
15.7468631623588));
#21699=CARTESIAN_POINT('Ctrl Pts',(-2.06363520780063,-0.505,15.7438749965183));
#21700=CARTESIAN_POINT('Ctrl Pts',(-1.93636479219937,-0.505,15.7438749965183));
#21701=CARTESIAN_POINT('Ctrl Pts',(-1.86863541965054,-0.492239912224197,
15.7468631623588));
#21702=CARTESIAN_POINT('Ctrl Pts',(-1.74427868605509,-0.440639774787125,
15.7575497283031));
#21703=CARTESIAN_POINT('Ctrl Pts',(-1.68763265613064,-0.401810505129054,
15.7650822805951));
#21704=CARTESIAN_POINT('Ctrl Pts',(-1.59819316383146,-0.312371012829873,
15.7791387482964));
#21705=CARTESIAN_POINT('Ctrl Pts',(-1.55936102475141,-0.255723435800378,
15.7865912587439));
#21706=CARTESIAN_POINT('Ctrl Pts',(-1.50775880152011,-0.131361285500179,
15.7970934401131));
#21707=CARTESIAN_POINT('Ctrl Pts',(-1.495,-0.0636299871652784,15.8));
#21708=CARTESIAN_POINT('Ctrl Pts',(-1.495,0.0636299871652782,15.8));
#21709=CARTESIAN_POINT('Ctrl Pts',(-1.50775880152011,0.131361285500179,
15.7970934401131));
#21710=CARTESIAN_POINT('Ctrl Pts',(-1.55936102475141,0.255723435800378,
15.7865912587439));
#21711=CARTESIAN_POINT('Ctrl Pts',(-1.59819316383146,0.312371012829873,
15.7791387482964));
#21712=CARTESIAN_POINT('Ctrl Pts',(-1.68763265613064,0.401810505129053,
15.7650822805951));
#21713=CARTESIAN_POINT('Ctrl Pts',(-1.74427868605509,0.440639774787125,
15.7575497283031));
#21714=CARTESIAN_POINT('Ctrl Pts',(-1.86863541965054,0.492239912224197,
15.7468631623588));
#21715=CARTESIAN_POINT('Ctrl Pts',(-1.93636479219937,0.505,15.7438749965183));
#21716=CARTESIAN_POINT('Ctrl Pts',(-2.,0.505,15.7438749965183));
#21717=CARTESIAN_POINT('',(-2.505,-6.18446633569413E-17,17.345));
#21718=CARTESIAN_POINT('',(-2.505,-6.18446633569413E-17,16.4725));
#21719=CARTESIAN_POINT('Origin',(-2.,0.,17.345));
#21720=CARTESIAN_POINT('Origin',(-2.,0.,17.3975));
#21721=CARTESIAN_POINT('',(-2.56,6.85802207522515E-17,17.4));
#21722=CARTESIAN_POINT('',(-2.5575,-6.82740590524649E-17,17.3975));
#21723=CARTESIAN_POINT('Origin',(-2.,0.,17.4));
#21724=CARTESIAN_POINT('Origin',(-6.2,-3.6,16.0783257246469));
#21725=CARTESIAN_POINT('',(-6.2,-3.6,15.9566514492938));
#21726=CARTESIAN_POINT('',(-6.2,-3.195,16.2));
#21727=CARTESIAN_POINT('',(-6.2,-3.3975,16.0783257246469));
#21728=CARTESIAN_POINT('Origin',(-6.2,-3.6,16.2));
#21729=CARTESIAN_POINT('Origin',(-6.2,-3.6,16.775));
#21730=CARTESIAN_POINT('',(-6.2,-3.195,16.3772771751247));
#21731=CARTESIAN_POINT('',(-6.2,-3.195,16.775));
#21732=CARTESIAN_POINT('',(-6.58891644346826,-3.487,16.682));
#21733=CARTESIAN_POINT('Ctrl Pts',(-6.58891644346826,-3.487,16.682));
#21734=CARTESIAN_POINT('Ctrl Pts',(-6.58891644346826,-3.487,16.6370619871072));
#21735=CARTESIAN_POINT('Ctrl Pts',(-6.58627670754491,-3.47639022136029,
16.5899241279869));
#21736=CARTESIAN_POINT('Ctrl Pts',(-6.57098354914856,-3.43610864188054,
16.5071507944627));
#21737=CARTESIAN_POINT('Ctrl Pts',(-6.55767741152601,-3.40643270490172,
16.471639261428));
#21738=CARTESIAN_POINT('Ctrl Pts',(-6.52737350118872,-3.36091702023246,
16.4342657910843));
#21739=CARTESIAN_POINT('Ctrl Pts',(-6.51499170641379,-3.34453211479069,
16.4232781228103));
#21740=CARTESIAN_POINT('Ctrl Pts',(-6.48629352194951,-3.31273768137677,
16.4058454179434));
#21741=CARTESIAN_POINT('Ctrl Pts',(-6.46996141031638,-3.29738179217064,
16.3993285535958));
#21742=CARTESIAN_POINT('Ctrl Pts',(-6.42036530129365,-3.25750827485252,
16.3851229200232));
#21743=CARTESIAN_POINT('Ctrl Pts',(-6.37932965869714,-3.23386275495577,
16.3810300297351));
#21744=CARTESIAN_POINT('Ctrl Pts',(-6.29109237758623,-3.20261126494113,
16.3772905860687));
#21745=CARTESIAN_POINT('Ctrl Pts',(-6.24390854386675,-3.195,16.3772771751247));
#21746=CARTESIAN_POINT('Ctrl Pts',(-6.2,-3.195,16.3772771751247));
#21747=CARTESIAN_POINT('',(-6.2,-3.195,16.9867228248753));
#21748=CARTESIAN_POINT('Ctrl Pts',(-6.2,-3.195,16.9867228248753));
#21749=CARTESIAN_POINT('Ctrl Pts',(-6.24390854386675,-3.195,16.9867228248753));
#21750=CARTESIAN_POINT('Ctrl Pts',(-6.29109237758623,-3.20261126494113,
16.9867094139313));
#21751=CARTESIAN_POINT('Ctrl Pts',(-6.37932965869714,-3.23386275495577,
16.9829699702649));
#21752=CARTESIAN_POINT('Ctrl Pts',(-6.42036530129365,-3.25750827485252,
16.9788770799768));
#21753=CARTESIAN_POINT('Ctrl Pts',(-6.46996141031638,-3.29738179217064,
16.9646714464042));
#21754=CARTESIAN_POINT('Ctrl Pts',(-6.48629352194951,-3.31273768137677,
16.9581545820566));
#21755=CARTESIAN_POINT('Ctrl Pts',(-6.51499170641379,-3.34453211479069,
16.9407218771897));
#21756=CARTESIAN_POINT('Ctrl Pts',(-6.52737350118872,-3.36091702023246,
16.9297342089157));
#21757=CARTESIAN_POINT('Ctrl Pts',(-6.55767741152601,-3.40643270490172,
16.892360738572));
#21758=CARTESIAN_POINT('Ctrl Pts',(-6.57098354914856,-3.43610864188054,
16.8568492055373));
#21759=CARTESIAN_POINT('Ctrl Pts',(-6.58627670754491,-3.47639022136029,
16.7740758720131));
#21760=CARTESIAN_POINT('Ctrl Pts',(-6.58891644346826,-3.487,16.7269380128928));
#21761=CARTESIAN_POINT('Ctrl Pts',(-6.58891644346826,-3.487,16.682));
#21762=CARTESIAN_POINT('',(-6.2,-3.195,17.35));
#21763=CARTESIAN_POINT('',(-6.2,-3.195,16.775));
#21764=CARTESIAN_POINT('Origin',(-6.2,-3.6,17.35));
#21765=CARTESIAN_POINT('Ctrl Pts',(-6.2,-3.195,16.3772771751247));
#21766=CARTESIAN_POINT('Ctrl Pts',(-6.15609145613325,-3.195,16.3772771751247));
#21767=CARTESIAN_POINT('Ctrl Pts',(-6.10890762241377,-3.20261126494113,
16.3772905860687));
#21768=CARTESIAN_POINT('Ctrl Pts',(-6.02067034130286,-3.23386275495577,
16.3810300297351));
#21769=CARTESIAN_POINT('Ctrl Pts',(-5.97963469870635,-3.25750827485252,
16.3851229200232));
#21770=CARTESIAN_POINT('Ctrl Pts',(-5.93003858968362,-3.29738179217064,
16.3993285535958));
#21771=CARTESIAN_POINT('Ctrl Pts',(-5.91370647805049,-3.31273768137677,
16.4058454179434));
#21772=CARTESIAN_POINT('Ctrl Pts',(-5.88500829358621,-3.34453211479069,
16.4232781228103));
#21773=CARTESIAN_POINT('Ctrl Pts',(-5.87262649881128,-3.36091702023246,
16.4342657910843));
#21774=CARTESIAN_POINT('Ctrl Pts',(-5.84232258847399,-3.40643270490172,
16.471639261428));
#21775=CARTESIAN_POINT('Ctrl Pts',(-5.82901645085144,-3.43610864188054,
16.5071507944627));
#21776=CARTESIAN_POINT('Ctrl Pts',(-5.81372329245509,-3.47639022136029,
16.5899241279869));
#21777=CARTESIAN_POINT('Ctrl Pts',(-5.81108355653174,-3.487,16.6370619871072));
#21778=CARTESIAN_POINT('Ctrl Pts',(-5.81108355653174,-3.487,16.682));
#21779=CARTESIAN_POINT('Ctrl Pts',(-5.81108355653174,-3.487,16.7269380128928));
#21780=CARTESIAN_POINT('Ctrl Pts',(-5.81372329245509,-3.47639022136029,
16.7740758720131));
#21781=CARTESIAN_POINT('Ctrl Pts',(-5.82901645085144,-3.43610864188054,
16.8568492055373));
#21782=CARTESIAN_POINT('Ctrl Pts',(-5.84232258847399,-3.40643270490172,
16.892360738572));
#21783=CARTESIAN_POINT('Ctrl Pts',(-5.87262649881128,-3.36091702023246,
16.9297342089157));
#21784=CARTESIAN_POINT('Ctrl Pts',(-5.88500829358621,-3.34453211479069,
16.9407218771897));
#21785=CARTESIAN_POINT('Ctrl Pts',(-5.91370647805049,-3.31273768137677,
16.9581545820566));
#21786=CARTESIAN_POINT('Ctrl Pts',(-5.93003858968362,-3.29738179217064,
16.9646714464042));
#21787=CARTESIAN_POINT('Ctrl Pts',(-5.97963469870635,-3.25750827485252,
16.9788770799768));
#21788=CARTESIAN_POINT('Ctrl Pts',(-6.02067034130286,-3.23386275495577,
16.9829699702649));
#21789=CARTESIAN_POINT('Ctrl Pts',(-6.10890762241377,-3.20261126494113,
16.9867094139313));
#21790=CARTESIAN_POINT('Ctrl Pts',(-6.15609145613325,-3.195,16.9867228248753));
#21791=CARTESIAN_POINT('Ctrl Pts',(-6.2,-3.195,16.9867228248753));
#21792=CARTESIAN_POINT('Origin',(-6.2,-3.6,17.4));
#21793=CARTESIAN_POINT('',(-6.2,-3.145,17.4));
#21794=CARTESIAN_POINT('',(-6.2,-3.145,17.4));
#21795=CARTESIAN_POINT('',(-6.6,-3.38314751557799,17.4));
#21796=CARTESIAN_POINT('Origin',(-6.2,-3.6,17.4));
#21797=CARTESIAN_POINT('',(-6.6,-3.81685248442201,17.4));
#21798=CARTESIAN_POINT('Ctrl Pts',(-6.60000000000001,-3.81685248442201,
17.4));
#21799=CARTESIAN_POINT('Ctrl Pts',(-6.60722705774228,-3.8035216567646,17.4));
#21800=CARTESIAN_POINT('Ctrl Pts',(-6.61371814969366,-3.78968189727386,
17.3998706495795));
#21801=CARTESIAN_POINT('Ctrl Pts',(-6.64208716999993,-3.71948476448862,
17.3989501445254));
#21802=CARTESIAN_POINT('Ctrl Pts',(-6.65268264098811,-3.6576935008072,17.3976826409881));
#21803=CARTESIAN_POINT('Ctrl Pts',(-6.65268264098811,-3.54039232396793,
17.3976826409881));
#21804=CARTESIAN_POINT('Ctrl Pts',(-6.64137663777292,-3.47668030239153,
17.3990538411799));
#21805=CARTESIAN_POINT('Ctrl Pts',(-6.61214628380182,-3.40699633192777,
17.3998996744314));
#21806=CARTESIAN_POINT('Ctrl Pts',(-6.60635819878554,-3.39487567041556,
17.4));
#21807=CARTESIAN_POINT('Ctrl Pts',(-6.6,-3.38314751557799,17.4));
#21808=CARTESIAN_POINT('Origin',(-6.2,-3.6,17.4));
#21809=CARTESIAN_POINT('Origin',(-7.2,0.,17.4));
#21810=CARTESIAN_POINT('',(-6.6,-4.6,17.4));
#21811=CARTESIAN_POINT('',(-6.6,0.,17.4));
#21812=CARTESIAN_POINT('',(6.6,-4.6,17.4));
#21813=CARTESIAN_POINT('',(7.2,-4.6,17.4));
#21814=CARTESIAN_POINT('',(6.6,-3.81685248442201,17.4));
#21815=CARTESIAN_POINT('',(6.6,0.,17.4));
#21816=CARTESIAN_POINT('',(6.2,-3.145,17.4));
#21817=CARTESIAN_POINT('Origin',(6.2,-3.6,17.4));
#21818=CARTESIAN_POINT('',(6.6,-3.38314751557799,17.4));
#21819=CARTESIAN_POINT('Origin',(6.2,-3.6,17.4));
#21820=CARTESIAN_POINT('',(6.6,3.38314751557798,17.4));
#21821=CARTESIAN_POINT('',(6.6,0.,17.4));
#21822=CARTESIAN_POINT('',(6.2,4.055,17.4));
#21823=CARTESIAN_POINT('Origin',(6.2,3.6,17.4));
#21824=CARTESIAN_POINT('',(6.6,3.81685248442202,17.4));
#21825=CARTESIAN_POINT('Origin',(6.2,3.6,17.4));
#21826=CARTESIAN_POINT('',(6.6,0.,17.4));
#21827=CARTESIAN_POINT('',(-6.6,3.81685248442202,17.4));
#21828=CARTESIAN_POINT('',(-6.6,0.,17.4));
#21829=CARTESIAN_POINT('',(-6.2,4.05500000000001,17.4));
#21830=CARTESIAN_POINT('Origin',(-6.2,3.6,17.4));
#21831=CARTESIAN_POINT('',(-6.6,3.38314751557798,17.4));
#21832=CARTESIAN_POINT('Origin',(-6.2,3.6,17.4));
#21833=CARTESIAN_POINT('',(-6.6,0.,17.4));
#21834=CARTESIAN_POINT('',(5.,-2.8,17.4));
#21835=CARTESIAN_POINT('',(-5.,-2.8,17.4));
#21836=CARTESIAN_POINT('',(-1.1,-2.8,17.4));
#21837=CARTESIAN_POINT('',(-5.,-2.4,17.4));
#21838=CARTESIAN_POINT('',(-5.,-1.4,17.4));
#21839=CARTESIAN_POINT('',(5.,-2.4,17.4));
#21840=CARTESIAN_POINT('',(-6.1,-2.4,17.4));
#21841=CARTESIAN_POINT('',(5.,-1.2,17.4));
#21842=CARTESIAN_POINT('',(5.,-1.2,17.4));
#21843=CARTESIAN_POINT('',(-5.,-1.2,17.4));
#21844=CARTESIAN_POINT('',(-1.1,-1.2,17.4));
#21845=CARTESIAN_POINT('',(-5.,-0.8,17.4));
#21846=CARTESIAN_POINT('',(-5.,-0.6,17.4));
#21847=CARTESIAN_POINT('',(5.,-0.8,17.4));
#21848=CARTESIAN_POINT('',(-6.1,-0.8,17.4));
#21849=CARTESIAN_POINT('',(5.,-0.4,17.4));
#21850=CARTESIAN_POINT('',(5.,2.4,17.4));
#21851=CARTESIAN_POINT('',(-5.,2.4,17.4));
#21852=CARTESIAN_POINT('',(-1.1,2.4,17.4));
#21853=CARTESIAN_POINT('',(-5.,2.8,17.4));
#21854=CARTESIAN_POINT('',(-5.,1.2,17.4));
#21855=CARTESIAN_POINT('',(5.,2.8,17.4));
#21856=CARTESIAN_POINT('',(-6.1,2.8,17.4));
#21857=CARTESIAN_POINT('',(5.,1.4,17.4));
#21858=CARTESIAN_POINT('',(5.,1.6,17.4));
#21859=CARTESIAN_POINT('',(-5.,1.6,17.4));
#21860=CARTESIAN_POINT('',(-1.1,1.6,17.4));
#21861=CARTESIAN_POINT('',(-5.,2.,17.4));
#21862=CARTESIAN_POINT('',(-5.,0.8,17.4));
#21863=CARTESIAN_POINT('',(5.,2.,17.4));
#21864=CARTESIAN_POINT('',(-6.1,2.,17.4));
#21865=CARTESIAN_POINT('',(5.,1.,17.4));
#21866=CARTESIAN_POINT('',(5.,0.8,17.4));
#21867=CARTESIAN_POINT('',(-5.,0.8,17.4));
#21868=CARTESIAN_POINT('',(-1.1,0.8,17.4));
#21869=CARTESIAN_POINT('',(-5.,1.2,17.4));
#21870=CARTESIAN_POINT('',(-5.,0.4,17.4));
#21871=CARTESIAN_POINT('',(5.,1.2,17.4));
#21872=CARTESIAN_POINT('',(-6.1,1.2,17.4));
#21873=CARTESIAN_POINT('',(5.,0.6,17.4));
#21874=CARTESIAN_POINT('',(5.,-2.,17.4));
#21875=CARTESIAN_POINT('',(-5.,-2.,17.4));
#21876=CARTESIAN_POINT('',(-1.1,-2.,17.4));
#21877=CARTESIAN_POINT('',(-5.,-1.6,17.4));
#21878=CARTESIAN_POINT('',(-5.,-1.,17.4));
#21879=CARTESIAN_POINT('',(5.,-1.6,17.4));
#21880=CARTESIAN_POINT('',(-6.1,-1.6,17.4));
#21881=CARTESIAN_POINT('',(5.,-0.8,17.4));
#21882=CARTESIAN_POINT('Origin',(-6.2,3.6,16.0783257246469));
#21883=CARTESIAN_POINT('',(-6.2,3.6,15.9566514492938));
#21884=CARTESIAN_POINT('',(-6.2,4.005,16.2));
#21885=CARTESIAN_POINT('',(-6.2,3.8025,16.0783257246469));
#21886=CARTESIAN_POINT('Origin',(-6.2,3.6,16.2));
#21887=CARTESIAN_POINT('Origin',(-6.2,3.6,16.775));
#21888=CARTESIAN_POINT('',(-6.2,4.005,17.35));
#21889=CARTESIAN_POINT('',(-6.2,4.005,16.775));
#21890=CARTESIAN_POINT('Origin',(-6.2,3.6,17.35));
#21891=CARTESIAN_POINT('',(-5.81108355653174,3.487,16.682));
#21892=CARTESIAN_POINT('',(-6.58891644346826,3.487,16.682));
#21893=CARTESIAN_POINT('Ctrl Pts',(-5.81108355653174,3.487,16.682));
#21894=CARTESIAN_POINT('Ctrl Pts',(-5.81108355653174,3.487,16.6370619871072));
#21895=CARTESIAN_POINT('Ctrl Pts',(-5.81372329245509,3.47639022136029,16.5899241279869));
#21896=CARTESIAN_POINT('Ctrl Pts',(-5.82901645085144,3.43610864188054,16.5071507944627));
#21897=CARTESIAN_POINT('Ctrl Pts',(-5.84232258847399,3.40643270490172,16.471639261428));
#21898=CARTESIAN_POINT('Ctrl Pts',(-5.87262649881128,3.36091702023246,16.4342657910843));
#21899=CARTESIAN_POINT('Ctrl Pts',(-5.88500829358621,3.34453211479069,16.4232781228103));
#21900=CARTESIAN_POINT('Ctrl Pts',(-5.91370647805049,3.31273768137677,16.4058454179434));
#21901=CARTESIAN_POINT('Ctrl Pts',(-5.93003858968362,3.29738179217064,16.3993285535958));
#21902=CARTESIAN_POINT('Ctrl Pts',(-5.97963469870635,3.25750827485252,16.3851229200232));
#21903=CARTESIAN_POINT('Ctrl Pts',(-6.02067034130286,3.23386275495577,16.3810300297351));
#21904=CARTESIAN_POINT('Ctrl Pts',(-6.10890762241377,3.20261126494113,16.3772905860687));
#21905=CARTESIAN_POINT('Ctrl Pts',(-6.15609145613325,3.195,16.3772771751247));
#21906=CARTESIAN_POINT('Ctrl Pts',(-6.24390854386675,3.195,16.3772771751247));
#21907=CARTESIAN_POINT('Ctrl Pts',(-6.29109237758623,3.20261126494113,16.3772905860687));
#21908=CARTESIAN_POINT('Ctrl Pts',(-6.37932965869714,3.23386275495577,16.3810300297351));
#21909=CARTESIAN_POINT('Ctrl Pts',(-6.42036530129365,3.25750827485252,16.3851229200232));
#21910=CARTESIAN_POINT('Ctrl Pts',(-6.46996141031638,3.29738179217064,16.3993285535958));
#21911=CARTESIAN_POINT('Ctrl Pts',(-6.48629352194951,3.31273768137677,16.4058454179434));
#21912=CARTESIAN_POINT('Ctrl Pts',(-6.51499170641379,3.34453211479069,16.4232781228103));
#21913=CARTESIAN_POINT('Ctrl Pts',(-6.52737350118872,3.36091702023246,16.4342657910843));
#21914=CARTESIAN_POINT('Ctrl Pts',(-6.55767741152601,3.40643270490172,16.471639261428));
#21915=CARTESIAN_POINT('Ctrl Pts',(-6.57098354914856,3.43610864188054,16.5071507944627));
#21916=CARTESIAN_POINT('Ctrl Pts',(-6.58627670754491,3.47639022136029,16.5899241279869));
#21917=CARTESIAN_POINT('Ctrl Pts',(-6.58891644346826,3.487,16.6370619871072));
#21918=CARTESIAN_POINT('Ctrl Pts',(-6.58891644346826,3.487,16.682));
#21919=CARTESIAN_POINT('Ctrl Pts',(-6.58891644346826,3.487,16.682));
#21920=CARTESIAN_POINT('Ctrl Pts',(-6.58891644346826,3.487,16.7269380128928));
#21921=CARTESIAN_POINT('Ctrl Pts',(-6.58627670754491,3.47639022136029,16.7740758720131));
#21922=CARTESIAN_POINT('Ctrl Pts',(-6.57098354914856,3.43610864188054,16.8568492055373));
#21923=CARTESIAN_POINT('Ctrl Pts',(-6.55767741152601,3.40643270490172,16.892360738572));
#21924=CARTESIAN_POINT('Ctrl Pts',(-6.52737350118872,3.36091702023246,16.9297342089157));
#21925=CARTESIAN_POINT('Ctrl Pts',(-6.51499170641379,3.34453211479069,16.9407218771897));
#21926=CARTESIAN_POINT('Ctrl Pts',(-6.48629352194951,3.31273768137677,16.9581545820566));
#21927=CARTESIAN_POINT('Ctrl Pts',(-6.46996141031638,3.29738179217064,16.9646714464042));
#21928=CARTESIAN_POINT('Ctrl Pts',(-6.42036530129365,3.25750827485252,16.9788770799768));
#21929=CARTESIAN_POINT('Ctrl Pts',(-6.37932965869714,3.23386275495577,16.9829699702649));
#21930=CARTESIAN_POINT('Ctrl Pts',(-6.29109237758623,3.20261126494113,16.9867094139313));
#21931=CARTESIAN_POINT('Ctrl Pts',(-6.24390854386675,3.195,16.9867228248753));
#21932=CARTESIAN_POINT('Ctrl Pts',(-6.15609145613325,3.195,16.9867228248753));
#21933=CARTESIAN_POINT('Ctrl Pts',(-6.10890762241377,3.20261126494113,16.9867094139313));
#21934=CARTESIAN_POINT('Ctrl Pts',(-6.02067034130286,3.23386275495577,16.9829699702649));
#21935=CARTESIAN_POINT('Ctrl Pts',(-5.97963469870635,3.25750827485252,16.9788770799768));
#21936=CARTESIAN_POINT('Ctrl Pts',(-5.93003858968362,3.29738179217064,16.9646714464042));
#21937=CARTESIAN_POINT('Ctrl Pts',(-5.91370647805049,3.31273768137677,16.9581545820566));
#21938=CARTESIAN_POINT('Ctrl Pts',(-5.88500829358621,3.34453211479069,16.9407218771897));
#21939=CARTESIAN_POINT('Ctrl Pts',(-5.87262649881128,3.36091702023246,16.9297342089157));
#21940=CARTESIAN_POINT('Ctrl Pts',(-5.84232258847399,3.40643270490172,16.892360738572));
#21941=CARTESIAN_POINT('Ctrl Pts',(-5.82901645085144,3.43610864188054,16.8568492055373));
#21942=CARTESIAN_POINT('Ctrl Pts',(-5.81372329245509,3.47639022136029,16.7740758720131));
#21943=CARTESIAN_POINT('Ctrl Pts',(-5.81108355653174,3.487,16.7269380128928));
#21944=CARTESIAN_POINT('Ctrl Pts',(-5.81108355653174,3.487,16.682));
#21945=CARTESIAN_POINT('Origin',(-6.2,3.6,17.4));
#21946=CARTESIAN_POINT('',(-6.2,4.055,17.4));
#21947=CARTESIAN_POINT('Ctrl Pts',(-6.6,3.38314751557798,17.4));
#21948=CARTESIAN_POINT('Ctrl Pts',(-6.60635819878554,3.39487567041556,17.4));
#21949=CARTESIAN_POINT('Ctrl Pts',(-6.61214628380182,3.40699633192776,17.3998996744314));
#21950=CARTESIAN_POINT('Ctrl Pts',(-6.64137663777293,3.47668030239153,17.3990538411799));
#21951=CARTESIAN_POINT('Ctrl Pts',(-6.65268264098811,3.54039232396793,17.3976826409881));
#21952=CARTESIAN_POINT('Ctrl Pts',(-6.65268264098811,3.6576935008072,17.3976826409881));
#21953=CARTESIAN_POINT('Ctrl Pts',(-6.64208716999993,3.71948476448862,17.3989501445254));
#21954=CARTESIAN_POINT('Ctrl Pts',(-6.61371814969366,3.78968189727386,17.3998706495795));
#21955=CARTESIAN_POINT('Ctrl Pts',(-6.60722705774228,3.80352165676461,17.4));
#21956=CARTESIAN_POINT('Ctrl Pts',(-6.6,3.81685248442202,17.4));
#21957=CARTESIAN_POINT('Origin',(-6.6,0.,16.8));
#21958=CARTESIAN_POINT('Ctrl Pts',(-7.2,3.51681487422156,16.8));
#21959=CARTESIAN_POINT('Ctrl Pts',(-7.2,3.51609674163657,16.8020376395857));
#21960=CARTESIAN_POINT('Ctrl Pts',(-7.19998961387021,3.5153556448834,16.8040498114376));
#21961=CARTESIAN_POINT('Ctrl Pts',(-7.19977035141354,3.50699129405166,16.8258511124764));
#21962=CARTESIAN_POINT('Ctrl Pts',(-7.19851062225153,3.49591868053171,16.8461520439008));
#21963=CARTESIAN_POINT('Ctrl Pts',(-7.19451004267811,3.46878210020379,16.8830829863768));
#21964=CARTESIAN_POINT('Ctrl Pts',(-7.19181581041583,3.45275112599972,16.8997422622249));
#21965=CARTESIAN_POINT('Ctrl Pts',(-7.1837030970831,3.40350950448746,16.9418791378472));
#21966=CARTESIAN_POINT('Ctrl Pts',(-7.17712501665467,3.36220580742002,16.9648485824245));
#21967=CARTESIAN_POINT('Ctrl Pts',(-7.16767615167579,3.27351018239752,16.9949156250641));
#21968=CARTESIAN_POINT('Ctrl Pts',(-7.16498109471003,3.22608873509771,17.00198109471));
#21969=CARTESIAN_POINT('Ctrl Pts',(-7.16498109471003,3.182,17.00198109471));
#21970=CARTESIAN_POINT('Ctrl Pts',(-7.16498109471003,3.13791126490229,17.00198109471));
#21971=CARTESIAN_POINT('Ctrl Pts',(-7.16767615167579,3.09048981760248,16.9949156250641));
#21972=CARTESIAN_POINT('Ctrl Pts',(-7.17712501665467,3.00179419257998,16.9648485824245));
#21973=CARTESIAN_POINT('Ctrl Pts',(-7.1837030970831,2.96049049551254,16.9418791378472));
#21974=CARTESIAN_POINT('Ctrl Pts',(-7.19181581041583,2.91124887400028,16.8997422622249));
#21975=CARTESIAN_POINT('Ctrl Pts',(-7.19451004267811,2.89521789979621,16.8830829863768));
#21976=CARTESIAN_POINT('Ctrl Pts',(-7.19851062225153,2.86808131946829,16.8461520439008));
#21977=CARTESIAN_POINT('Ctrl Pts',(-7.19977035141354,2.85700870594834,16.8258511124764));
#21978=CARTESIAN_POINT('Ctrl Pts',(-7.19998961387021,2.8486443551166,16.8040498114376));
#21979=CARTESIAN_POINT('Ctrl Pts',(-7.2,2.84790325836343,16.8020376395857));
#21980=CARTESIAN_POINT('Ctrl Pts',(-7.2,2.84718512577844,16.8));
#21981=CARTESIAN_POINT('Ctrl Pts',(-7.2,-2.84718512577844,16.8));
#21982=CARTESIAN_POINT('Ctrl Pts',(-7.2,-2.84790325836343,16.8020376395857));
#21983=CARTESIAN_POINT('Ctrl Pts',(-7.19998961387021,-2.8486443551166,16.8040498114376));
#21984=CARTESIAN_POINT('Ctrl Pts',(-7.19977035141354,-2.85700870594834,
16.8258511124764));
#21985=CARTESIAN_POINT('Ctrl Pts',(-7.19851062225153,-2.86808131946829,
16.8461520439008));
#21986=CARTESIAN_POINT('Ctrl Pts',(-7.19451004267811,-2.89521789979621,
16.8830829863768));
#21987=CARTESIAN_POINT('Ctrl Pts',(-7.19181581041583,-2.91124887400028,
16.8997422622249));
#21988=CARTESIAN_POINT('Ctrl Pts',(-7.1837030970831,-2.96049049551254,16.9418791378472));
#21989=CARTESIAN_POINT('Ctrl Pts',(-7.17712501665467,-3.00179419257999,
16.9648485824245));
#21990=CARTESIAN_POINT('Ctrl Pts',(-7.16767615167579,-3.09048981760248,
16.9949156250641));
#21991=CARTESIAN_POINT('Ctrl Pts',(-7.16498109471003,-3.13791126490229,
17.00198109471));
#21992=CARTESIAN_POINT('Ctrl Pts',(-7.16498109471003,-3.182,17.00198109471));
#21993=CARTESIAN_POINT('Ctrl Pts',(-7.16498109471003,-3.22608873509771,
17.00198109471));
#21994=CARTESIAN_POINT('Ctrl Pts',(-7.16767615167579,-3.27351018239752,
16.9949156250641));
#21995=CARTESIAN_POINT('Ctrl Pts',(-7.17712501665467,-3.36220580742002,
16.9648485824245));
#21996=CARTESIAN_POINT('Ctrl Pts',(-7.1837030970831,-3.40350950448746,16.9418791378472));
#21997=CARTESIAN_POINT('Ctrl Pts',(-7.19181581041583,-3.45275112599972,
16.8997422622249));
#21998=CARTESIAN_POINT('Ctrl Pts',(-7.19451004267811,-3.46878210020379,
16.8830829863768));
#21999=CARTESIAN_POINT('Ctrl Pts',(-7.19851062225153,-3.49591868053171,
16.8461520439008));
#22000=CARTESIAN_POINT('Ctrl Pts',(-7.19977035141354,-3.50699129405166,
16.8258511124764));
#22001=CARTESIAN_POINT('Ctrl Pts',(-7.19998961387021,-3.5153556448834,16.8040498114376));
#22002=CARTESIAN_POINT('Ctrl Pts',(-7.2,-3.51609674163657,16.8020376395857));
#22003=CARTESIAN_POINT('Ctrl Pts',(-7.2,-3.51681487422156,16.8));
#22004=CARTESIAN_POINT('Origin',(-6.6,-4.6,16.8));
#22005=CARTESIAN_POINT('Origin',(6.2,-3.6,16.0783257246469));
#22006=CARTESIAN_POINT('',(6.2,-3.6,15.9566514492938));
#22007=CARTESIAN_POINT('',(6.2,-3.195,16.2));
#22008=CARTESIAN_POINT('',(6.2,-3.3975,16.0783257246469));
#22009=CARTESIAN_POINT('Origin',(6.2,-3.6,16.2));
#22010=CARTESIAN_POINT('Origin',(6.2,-3.6,16.775));
#22011=CARTESIAN_POINT('',(6.2,-3.195,17.35));
#22012=CARTESIAN_POINT('',(6.2,-3.195,16.775));
#22013=CARTESIAN_POINT('Origin',(6.2,-3.6,17.35));
#22014=CARTESIAN_POINT('Origin',(6.2,-3.6,17.4));
#22015=CARTESIAN_POINT('',(6.2,-3.145,17.4));
#22016=CARTESIAN_POINT('Ctrl Pts',(6.6,-3.38314751557799,17.4));
#22017=CARTESIAN_POINT('Ctrl Pts',(6.60635819878554,-3.39487567041556,17.4));
#22018=CARTESIAN_POINT('Ctrl Pts',(6.61214628380182,-3.40699633192777,17.3998996744314));
#22019=CARTESIAN_POINT('Ctrl Pts',(6.64137663777292,-3.47668030239153,17.3990538411799));
#22020=CARTESIAN_POINT('Ctrl Pts',(6.65268264098811,-3.54039232396793,17.3976826409881));
#22021=CARTESIAN_POINT('Ctrl Pts',(6.65268264098811,-3.6576935008072,17.3976826409881));
#22022=CARTESIAN_POINT('Ctrl Pts',(6.64208716999993,-3.71948476448862,17.3989501445254));
#22023=CARTESIAN_POINT('Ctrl Pts',(6.61371814969366,-3.78968189727386,17.3998706495795));
#22024=CARTESIAN_POINT('Ctrl Pts',(6.60722705774228,-3.8035216567646,17.4));
#22025=CARTESIAN_POINT('Ctrl Pts',(6.6,-3.81685248442201,17.4));
#22026=CARTESIAN_POINT('Origin',(6.6,0.,16.8));
#22027=CARTESIAN_POINT('Origin',(6.6,-4.6,16.8));
#22028=CARTESIAN_POINT('Ctrl Pts',(6.6,3.81685248442202,17.4));
#22029=CARTESIAN_POINT('Ctrl Pts',(6.60722705774228,3.80352165676461,17.4));
#22030=CARTESIAN_POINT('Ctrl Pts',(6.61371814969366,3.78968189727386,17.3998706495795));
#22031=CARTESIAN_POINT('Ctrl Pts',(6.64208716999993,3.71948476448862,17.3989501445254));
#22032=CARTESIAN_POINT('Ctrl Pts',(6.65268264098811,3.6576935008072,17.3976826409881));
#22033=CARTESIAN_POINT('Ctrl Pts',(6.65268264098811,3.54039232396793,17.3976826409881));
#22034=CARTESIAN_POINT('Ctrl Pts',(6.64137663777293,3.47668030239153,17.3990538411799));
#22035=CARTESIAN_POINT('Ctrl Pts',(6.61214628380182,3.40699633192776,17.3998996744314));
#22036=CARTESIAN_POINT('Ctrl Pts',(6.60635819878554,3.39487567041556,17.4));
#22037=CARTESIAN_POINT('Ctrl Pts',(6.6,3.38314751557798,17.4));
#22038=CARTESIAN_POINT('Origin',(6.2,3.6,16.0783257246469));
#22039=CARTESIAN_POINT('',(6.2,3.6,15.9566514492938));
#22040=CARTESIAN_POINT('',(6.2,4.005,16.2));
#22041=CARTESIAN_POINT('',(6.2,3.8025,16.0783257246469));
#22042=CARTESIAN_POINT('Origin',(6.2,3.6,16.2));
#22043=CARTESIAN_POINT('Origin',(6.2,3.6,16.775));
#22044=CARTESIAN_POINT('',(6.2,4.005,17.35));
#22045=CARTESIAN_POINT('',(6.2,4.005,16.775));
#22046=CARTESIAN_POINT('Origin',(6.2,3.6,17.35));
#22047=CARTESIAN_POINT('Origin',(6.2,3.6,17.4));
#22048=CARTESIAN_POINT('',(6.2,4.055,17.4));
#22049=CARTESIAN_POINT('Origin',(-4.,4.3083687555983,2.6));
#22050=CARTESIAN_POINT('',(-4.,4.21673751119659,2.6));
#22051=CARTESIAN_POINT('',(-3.695,4.4,2.6));
#22052=CARTESIAN_POINT('',(-3.8475,4.3083687555983,2.6));
#22053=CARTESIAN_POINT('Origin',(-4.,4.4,2.6));
#22054=CARTESIAN_POINT('Origin',(-4.,4.975,2.6));
#22055=CARTESIAN_POINT('',(-3.695,5.55,2.6));
#22056=CARTESIAN_POINT('',(-3.695,4.975,2.6));
#22057=CARTESIAN_POINT('Origin',(-4.,5.55,2.6));
#22058=CARTESIAN_POINT('Origin',(-4.,5.6,2.6));
#22059=CARTESIAN_POINT('',(-3.645,5.6,2.6));
#22060=CARTESIAN_POINT('Origin',(-4.,-2.7083687555983,2.6));
#22061=CARTESIAN_POINT('',(-4.,-2.61673751119659,2.6));
#22062=CARTESIAN_POINT('',(-4.305,-2.8,2.6));
#22063=CARTESIAN_POINT('',(-4.1525,-2.7083687555983,2.6));
#22064=CARTESIAN_POINT('Origin',(-4.,-2.8,2.6));
#22065=CARTESIAN_POINT('Origin',(-4.,-3.675,2.6));
#22066=CARTESIAN_POINT('',(-4.305,-4.55,2.6));
#22067=CARTESIAN_POINT('',(-4.305,-3.675,2.6));
#22068=CARTESIAN_POINT('Origin',(-4.,-4.55,2.6));
#22069=CARTESIAN_POINT('Origin',(-4.,-4.6,2.6));
#22070=CARTESIAN_POINT('',(-4.355,-4.6,2.6));
#22071=CARTESIAN_POINT('',(-4.355,-4.6,2.6));
#22072=CARTESIAN_POINT('Origin',(-4.,-4.6,2.6));
#22073=CARTESIAN_POINT('Origin',(4.,4.3083687555983,2.6));
#22074=CARTESIAN_POINT('',(4.,4.21673751119659,2.6));
#22075=CARTESIAN_POINT('',(4.305,4.4,2.6));
#22076=CARTESIAN_POINT('',(4.1525,4.3083687555983,2.6));
#22077=CARTESIAN_POINT('Origin',(4.,4.4,2.6));
#22078=CARTESIAN_POINT('Origin',(4.,4.975,2.6));
#22079=CARTESIAN_POINT('',(4.305,5.55,2.6));
#22080=CARTESIAN_POINT('',(4.305,4.975,2.6));
#22081=CARTESIAN_POINT('Origin',(4.,5.55,2.6));
#22082=CARTESIAN_POINT('Origin',(4.,5.6,2.6));
#22083=CARTESIAN_POINT('',(4.355,5.6,2.6));
#22084=CARTESIAN_POINT('Origin',(4.,-2.7083687555983,2.6));
#22085=CARTESIAN_POINT('',(4.,-2.61673751119659,2.6));
#22086=CARTESIAN_POINT('',(3.695,-2.8,2.6));
#22087=CARTESIAN_POINT('',(3.8475,-2.7083687555983,2.6));
#22088=CARTESIAN_POINT('Origin',(4.,-2.8,2.6));
#22089=CARTESIAN_POINT('Origin',(4.,-3.675,2.6));
#22090=CARTESIAN_POINT('',(3.695,-4.55,2.6));
#22091=CARTESIAN_POINT('',(3.695,-3.675,2.6));
#22092=CARTESIAN_POINT('Origin',(4.,-4.55,2.6));
#22093=CARTESIAN_POINT('Origin',(4.,-4.6,2.6));
#22094=CARTESIAN_POINT('',(3.645,-4.6,2.6));
#22095=CARTESIAN_POINT('',(3.645,-4.6,2.6));
#22096=CARTESIAN_POINT('Origin',(4.,-4.6,2.6));
#22097=CARTESIAN_POINT('Origin',(-6.,4.3083687555983,8.));
#22098=CARTESIAN_POINT('',(-6.,4.21673751119659,8.));
#22099=CARTESIAN_POINT('',(-5.695,4.4,8.));
#22100=CARTESIAN_POINT('',(-5.8475,4.3083687555983,8.));
#22101=CARTESIAN_POINT('Origin',(-6.,4.4,8.));
#22102=CARTESIAN_POINT('Origin',(-6.,4.975,8.));
#22103=CARTESIAN_POINT('',(-5.695,5.55,8.));
#22104=CARTESIAN_POINT('',(-5.695,4.975,8.));
#22105=CARTESIAN_POINT('Origin',(-6.,5.55,8.));
#22106=CARTESIAN_POINT('Origin',(-6.,5.6,8.));
#22107=CARTESIAN_POINT('',(-5.645,5.6,8.));
#22108=CARTESIAN_POINT('Origin',(-6.,-2.7083687555983,8.));
#22109=CARTESIAN_POINT('',(-6.,-2.61673751119659,8.));
#22110=CARTESIAN_POINT('',(-6.305,-2.8,8.));
#22111=CARTESIAN_POINT('',(-6.1525,-2.7083687555983,8.));
#22112=CARTESIAN_POINT('Origin',(-6.,-2.8,8.));
#22113=CARTESIAN_POINT('Origin',(-6.,-3.675,8.));
#22114=CARTESIAN_POINT('',(-6.305,-4.55,8.));
#22115=CARTESIAN_POINT('',(-6.305,-3.675,8.));
#22116=CARTESIAN_POINT('Origin',(-6.,-4.55,8.));
#22117=CARTESIAN_POINT('Origin',(-6.,-4.6,8.));
#22118=CARTESIAN_POINT('',(-6.355,-4.6,8.));
#22119=CARTESIAN_POINT('',(-6.355,-4.6,8.));
#22120=CARTESIAN_POINT('Origin',(-6.,-4.6,8.));
#22121=CARTESIAN_POINT('Origin',(6.,4.3083687555983,8.));
#22122=CARTESIAN_POINT('',(6.,4.21673751119659,8.));
#22123=CARTESIAN_POINT('',(6.305,4.4,8.));
#22124=CARTESIAN_POINT('',(6.1525,4.3083687555983,8.));
#22125=CARTESIAN_POINT('Origin',(6.,4.4,8.));
#22126=CARTESIAN_POINT('Origin',(6.,4.975,8.));
#22127=CARTESIAN_POINT('',(6.305,5.55,8.));
#22128=CARTESIAN_POINT('',(6.305,4.975,8.));
#22129=CARTESIAN_POINT('Origin',(6.,5.55,8.));
#22130=CARTESIAN_POINT('Origin',(6.,5.6,8.));
#22131=CARTESIAN_POINT('',(6.355,5.6,8.));
#22132=CARTESIAN_POINT('Origin',(6.,-2.7083687555983,8.));
#22133=CARTESIAN_POINT('',(6.,-2.61673751119659,8.));
#22134=CARTESIAN_POINT('',(5.695,-2.8,8.));
#22135=CARTESIAN_POINT('',(5.8475,-2.7083687555983,8.));
#22136=CARTESIAN_POINT('Origin',(6.,-2.8,8.));
#22137=CARTESIAN_POINT('Origin',(6.,-3.675,8.));
#22138=CARTESIAN_POINT('',(5.695,-4.55,8.));
#22139=CARTESIAN_POINT('',(5.695,-3.675,8.));
#22140=CARTESIAN_POINT('Origin',(6.,-4.55,8.));
#22141=CARTESIAN_POINT('Origin',(6.,-4.6,8.));
#22142=CARTESIAN_POINT('',(5.645,-4.6,8.));
#22143=CARTESIAN_POINT('',(5.645,-4.6,8.));
#22144=CARTESIAN_POINT('Origin',(6.,-4.6,8.));
#22145=CARTESIAN_POINT('Origin',(-5.3083687555983,-3.182,10.318));
#22146=CARTESIAN_POINT('',(-5.21673751119659,-3.182,10.318));
#22147=CARTESIAN_POINT('',(-5.4,-2.877,10.318));
#22148=CARTESIAN_POINT('',(-5.3083687555983,-3.0295,10.318));
#22149=CARTESIAN_POINT('Origin',(-5.4,-3.182,10.318));
#22150=CARTESIAN_POINT('Origin',(-6.275,-3.182,10.318));
#22151=CARTESIAN_POINT('',(-7.15,-2.877,10.318));
#22152=CARTESIAN_POINT('',(-6.275,-2.877,10.318));
#22153=CARTESIAN_POINT('Origin',(-7.15,-3.182,10.318));
#22154=CARTESIAN_POINT('Origin',(-7.2,-3.182,10.318));
#22155=CARTESIAN_POINT('',(-7.2,-2.827,10.318));
#22156=CARTESIAN_POINT('Origin',(-5.3083687555983,3.182,10.318));
#22157=CARTESIAN_POINT('',(-5.21673751119659,3.182,10.318));
#22158=CARTESIAN_POINT('',(-5.4,3.487,10.318));
#22159=CARTESIAN_POINT('',(-5.3083687555983,3.3345,10.318));
#22160=CARTESIAN_POINT('Origin',(-5.4,3.182,10.318));
#22161=CARTESIAN_POINT('Origin',(-6.275,3.182,10.318));
#22162=CARTESIAN_POINT('',(-7.15,3.487,10.318));
#22163=CARTESIAN_POINT('',(-6.275,3.487,10.318));
#22164=CARTESIAN_POINT('Origin',(-7.15,3.182,10.318));
#22165=CARTESIAN_POINT('Origin',(-7.2,3.182,10.318));
#22166=CARTESIAN_POINT('',(-7.2,3.537,10.318));
#22167=CARTESIAN_POINT('Origin',(-5.3083687555983,-3.182,16.682));
#22168=CARTESIAN_POINT('',(-5.21673751119659,-3.182,16.682));
#22169=CARTESIAN_POINT('',(-5.4,-2.877,16.682));
#22170=CARTESIAN_POINT('',(-5.3083687555983,-3.0295,16.682));
#22171=CARTESIAN_POINT('Origin',(-5.4,-3.182,16.682));
#22172=CARTESIAN_POINT('Origin',(-6.275,-3.182,16.682));
#22173=CARTESIAN_POINT('',(-7.15,-2.877,16.682));
#22174=CARTESIAN_POINT('',(-6.275,-2.877,16.682));
#22175=CARTESIAN_POINT('Origin',(-7.15,-3.182,16.682));
#22176=CARTESIAN_POINT('Origin',(-7.2,-3.182,16.682));
#22177=CARTESIAN_POINT('',(-7.2,-2.827,16.682));
#22178=CARTESIAN_POINT('Origin',(-5.3083687555983,3.182,16.682));
#22179=CARTESIAN_POINT('',(-5.21673751119659,3.182,16.682));
#22180=CARTESIAN_POINT('',(-5.4,3.487,16.682));
#22181=CARTESIAN_POINT('',(-5.3083687555983,3.3345,16.682));
#22182=CARTESIAN_POINT('Origin',(-5.4,3.182,16.682));
#22183=CARTESIAN_POINT('Origin',(-6.275,3.182,16.682));
#22184=CARTESIAN_POINT('',(-6.275,3.487,16.682));
#22185=CARTESIAN_POINT('',(-7.15,3.487,16.682));
#22186=CARTESIAN_POINT('',(-6.275,3.487,16.682));
#22187=CARTESIAN_POINT('Origin',(-7.15,3.182,16.682));
#22188=CARTESIAN_POINT('Origin',(-7.2,3.182,16.682));
#22189=CARTESIAN_POINT('',(-7.2,3.537,16.682));
#22190=CARTESIAN_POINT('Origin',(-6.,-4.1,0.6375));
#22191=CARTESIAN_POINT('',(-6.,-4.525,1.2));
#22192=CARTESIAN_POINT('Origin',(-6.,-4.1,1.2));
#22193=CARTESIAN_POINT('',(-6.,-4.525,0.025));
#22194=CARTESIAN_POINT('',(-6.,-4.525,0.6375));
#22195=CARTESIAN_POINT('Origin',(-6.,-4.1,0.025));
#22196=CARTESIAN_POINT('Origin',(-6.,-4.1,-0.0125));
#22197=CARTESIAN_POINT('',(-6.,-4.55,0.));
#22198=CARTESIAN_POINT('',(-6.,-4.5625,-0.0125));
#22199=CARTESIAN_POINT('Origin',(-6.,-4.1,0.));
#22200=CARTESIAN_POINT('Origin',(-6.,4.1,0.6375));
#22201=CARTESIAN_POINT('',(-6.,3.675,1.2));
#22202=CARTESIAN_POINT('Origin',(-6.,4.1,1.2));
#22203=CARTESIAN_POINT('',(-6.,3.675,0.025));
#22204=CARTESIAN_POINT('',(-6.,3.675,0.6375));
#22205=CARTESIAN_POINT('Origin',(-6.,4.1,0.025));
#22206=CARTESIAN_POINT('Origin',(-6.,4.1,-0.0125));
#22207=CARTESIAN_POINT('',(-6.,3.65,0.));
#22208=CARTESIAN_POINT('',(-6.,3.6375,-0.0125));
#22209=CARTESIAN_POINT('Origin',(-6.,4.1,0.));
#22210=CARTESIAN_POINT('Origin',(6.,-4.1,0.6375));
#22211=CARTESIAN_POINT('',(6.,-4.525,1.2));
#22212=CARTESIAN_POINT('Origin',(6.,-4.1,1.2));
#22213=CARTESIAN_POINT('',(6.,-4.525,0.025));
#22214=CARTESIAN_POINT('',(6.,-4.525,0.6375));
#22215=CARTESIAN_POINT('Origin',(6.,-4.1,0.025));
#22216=CARTESIAN_POINT('Origin',(6.,-4.1,-0.0125));
#22217=CARTESIAN_POINT('',(6.,-4.55,0.));
#22218=CARTESIAN_POINT('',(6.,-4.5625,-0.0125));
#22219=CARTESIAN_POINT('Origin',(6.,-4.1,0.));
#22220=CARTESIAN_POINT('Origin',(6.,4.1,0.6375));
#22221=CARTESIAN_POINT('',(6.,3.675,1.2));
#22222=CARTESIAN_POINT('Origin',(6.,4.1,1.2));
#22223=CARTESIAN_POINT('',(6.,3.675,0.025));
#22224=CARTESIAN_POINT('',(6.,3.675,0.6375));
#22225=CARTESIAN_POINT('Origin',(6.,4.1,0.025));
#22226=CARTESIAN_POINT('Origin',(6.,4.1,-0.0125));
#22227=CARTESIAN_POINT('',(6.,3.65,0.));
#22228=CARTESIAN_POINT('',(6.,3.6375,-0.0125));
#22229=CARTESIAN_POINT('Origin',(6.,4.1,0.));
#22230=CARTESIAN_POINT('Origin',(4.8,-3.6,3.4));
#22231=CARTESIAN_POINT('',(4.8,-4.6,1.2));
#22232=CARTESIAN_POINT('',(4.8,-4.6,6.05));
#22233=CARTESIAN_POINT('',(4.8,-3.6,1.2));
#22234=CARTESIAN_POINT('Origin',(4.8,-3.6,1.2));
#22235=CARTESIAN_POINT('',(2.4,-4.6,1.2));
#22236=CARTESIAN_POINT('Origin',(-4.8,-3.6,3.4));
#22237=CARTESIAN_POINT('',(-4.8,-4.6,3.4));
#22238=CARTESIAN_POINT('',(-4.8,-3.6,3.4));
#22239=CARTESIAN_POINT('',(-2.4,-4.6,3.4));
#22240=CARTESIAN_POINT('Origin',(-4.8,-3.6,1.2));
#22241=CARTESIAN_POINT('',(-4.8,-4.6,1.2));
#22242=CARTESIAN_POINT('',(-4.8,-4.6,4.95));
#22243=CARTESIAN_POINT('',(-4.8,-3.6,1.2));
#22244=CARTESIAN_POINT('Origin',(-7.3,-3.6,1.2));
#22245=CARTESIAN_POINT('',(-3.65,-4.6,1.2));
#22246=CARTESIAN_POINT('Origin',(0.,-4.6,8.7));
#22247=CARTESIAN_POINT('',(-6.6,-4.6,0.));
#22248=CARTESIAN_POINT('Origin',(-6.6,-4.6,0.6));
#22249=CARTESIAN_POINT('',(-4.,-4.6,0.));
#22250=CARTESIAN_POINT('',(-7.2,-4.6,0.));
#22251=CARTESIAN_POINT('',(-4.,-4.6,0.8));
#22252=CARTESIAN_POINT('',(-4.,-4.6,4.3));
#22253=CARTESIAN_POINT('',(4.,-4.6,0.8));
#22254=CARTESIAN_POINT('',(-2.,-4.6,0.8));
#22255=CARTESIAN_POINT('',(4.,-4.6,0.));
#22256=CARTESIAN_POINT('',(4.,-4.6,4.75));
#22257=CARTESIAN_POINT('',(6.6,-4.6,0.));
#22258=CARTESIAN_POINT('',(-7.2,-4.6,0.));
#22259=CARTESIAN_POINT('Origin',(6.6,-4.6,0.6));
#22260=CARTESIAN_POINT('',(-6.49062803548097E-16,-4.6,1.9));
#22261=CARTESIAN_POINT('Origin',(0.,-4.6,7.2));
#22262=CARTESIAN_POINT('Origin',(7.3,3.6,1.2));
#22263=CARTESIAN_POINT('',(4.8,4.6,1.2));
#22264=CARTESIAN_POINT('',(3.65,4.6,1.2));
#22265=CARTESIAN_POINT('',(4.8,3.6,1.2));
#22266=CARTESIAN_POINT('',(4.8,3.6,1.2));
#22267=CARTESIAN_POINT('',(4.8,3.6,1.2));
#22268=CARTESIAN_POINT('Origin',(6.05,3.6,2.3));
#22269=CARTESIAN_POINT('',(4.8,3.6,3.4));
#22270=CARTESIAN_POINT('',(4.8,3.6,3.4));
#22271=CARTESIAN_POINT('',(7.3,3.6,3.4));
#22272=CARTESIAN_POINT('Origin',(4.8,3.6,1.2));
#22273=CARTESIAN_POINT('',(4.8,3.6,3.4));
#22274=CARTESIAN_POINT('',(4.8,4.6,2.18768943743823));
#22275=CARTESIAN_POINT('',(4.8,4.6,4.95));
#22276=CARTESIAN_POINT('',(4.8,4.6,2.18768943743823));
#22277=CARTESIAN_POINT('Origin',(4.8,3.6,3.4));
#22278=CARTESIAN_POINT('Origin',(-4.8,3.6,3.4));
#22279=CARTESIAN_POINT('',(-4.8,4.6,2.18768943743823));
#22280=CARTESIAN_POINT('',(-4.8,4.6,2.18768943743823));
#22281=CARTESIAN_POINT('',(-4.8,4.6,1.2));
#22282=CARTESIAN_POINT('',(-4.8,4.6,6.05));
#22283=CARTESIAN_POINT('',(-4.8,3.6,1.2));
#22284=CARTESIAN_POINT('',(-4.8,3.6,1.2));
#22285=CARTESIAN_POINT('',(-4.8,3.6,1.2));
#22286=CARTESIAN_POINT('',(-4.8,4.6,3.01231056256177));
#22287=CARTESIAN_POINT('Origin',(-4.8,3.6,1.2));
#22288=CARTESIAN_POINT('',(-2.4,4.6,1.2));
#22289=CARTESIAN_POINT('',(-7.3,3.6,1.2));
#22290=CARTESIAN_POINT('Origin',(-6.05,3.6,2.3));
#22291=CARTESIAN_POINT('Origin',(4.,4.6,2.6));
#22292=CARTESIAN_POINT('',(3.14292474054464,4.6,2.32536933960403));
#22293=CARTESIAN_POINT('Origin',(4.,4.6,2.6));
#22294=CARTESIAN_POINT('',(3.14292474054464,4.6,2.32536933960403));
#22295=CARTESIAN_POINT('Origin',(-4.,4.6,2.6));
#22296=CARTESIAN_POINT('Origin',(-4.,4.6,2.6));
#22297=CARTESIAN_POINT('',(-3.14292474054464,4.6,2.32536933960403));
#22298=CARTESIAN_POINT('',(-3.14292474054464,4.6,2.32536933960403));
#22299=CARTESIAN_POINT('Origin',(-4.,4.6,2.6));
#22300=CARTESIAN_POINT('Origin',(0.,4.6,8.7));
#22301=CARTESIAN_POINT('',(6.6,4.6,0.));
#22302=CARTESIAN_POINT('Origin',(6.6,4.6,0.6));
#22303=CARTESIAN_POINT('',(4.,4.6,0.));
#22304=CARTESIAN_POINT('',(-7.2,4.6,0.));
#22305=CARTESIAN_POINT('',(4.,4.6,0.8));
#22306=CARTESIAN_POINT('',(4.,4.6,4.75));
#22307=CARTESIAN_POINT('',(-4.,4.6,0.8));
#22308=CARTESIAN_POINT('',(-2.,4.6,0.8));
#22309=CARTESIAN_POINT('',(-4.,4.6,0.));
#22310=CARTESIAN_POINT('',(-4.,4.6,4.3));
#22311=CARTESIAN_POINT('',(-6.6,4.6,0.));
#22312=CARTESIAN_POINT('',(-7.2,4.6,0.));
#22313=CARTESIAN_POINT('Origin',(-6.6,4.6,0.6));
#22314=CARTESIAN_POINT('Origin',(0.,4.6,7.2));
#22315=CARTESIAN_POINT('Origin',(-4.,0.,-0.1));
#22316=CARTESIAN_POINT('',(-4.,0.,0.8));
#22317=CARTESIAN_POINT('',(-4.,0.,0.));
#22318=CARTESIAN_POINT('Origin',(4.,0.,0.8));
#22319=CARTESIAN_POINT('',(4.,0.,0.));
#22320=CARTESIAN_POINT('',(4.,0.,0.8));
#22321=CARTESIAN_POINT('Origin',(-4.,0.,0.8));
#22322=CARTESIAN_POINT('Origin',(7.2,0.,0.));
#22323=CARTESIAN_POINT('',(6.6,0.,0.));
#22324=CARTESIAN_POINT('Origin',(7.2,0.,0.));
#22325=CARTESIAN_POINT('',(-6.6,0.,0.));
#22326=CARTESIAN_POINT('Origin',(5.,-2.,17.4));
#22327=CARTESIAN_POINT('',(5.,-2.,16.6));
#22328=CARTESIAN_POINT('',(5.,-2.,17.4));
#22329=CARTESIAN_POINT('',(-5.,-2.,16.6));
#22330=CARTESIAN_POINT('',(-5.,-2.,16.6));
#22331=CARTESIAN_POINT('',(-5.,-2.,17.4));
#22332=CARTESIAN_POINT('Origin',(5.,-1.6,17.4));
#22333=CARTESIAN_POINT('',(5.,-1.6,16.6));
#22334=CARTESIAN_POINT('',(5.,-1.6,17.4));
#22335=CARTESIAN_POINT('',(5.,-2.,16.6));
#22336=CARTESIAN_POINT('Origin',(-5.,-1.6,17.4));
#22337=CARTESIAN_POINT('',(-5.,-1.6,16.6));
#22338=CARTESIAN_POINT('',(-5.,-1.6,17.4));
#22339=CARTESIAN_POINT('',(5.,-1.6,16.6));
#22340=CARTESIAN_POINT('Origin',(-5.,-2.,17.4));
#22341=CARTESIAN_POINT('',(-5.,-1.6,16.6));
#22342=CARTESIAN_POINT('Origin',(0.,-1.8,16.6));
#22343=CARTESIAN_POINT('Origin',(5.,0.8,17.4));
#22344=CARTESIAN_POINT('',(5.,0.8,16.6));
#22345=CARTESIAN_POINT('',(5.,0.8,17.4));
#22346=CARTESIAN_POINT('',(-5.,0.8,16.6));
#22347=CARTESIAN_POINT('',(-5.,0.8,16.6));
#22348=CARTESIAN_POINT('',(-5.,0.8,17.4));
#22349=CARTESIAN_POINT('Origin',(5.,1.2,17.4));
#22350=CARTESIAN_POINT('',(5.,1.2,16.6));
#22351=CARTESIAN_POINT('',(5.,1.2,17.4));
#22352=CARTESIAN_POINT('',(5.,0.8,16.6));
#22353=CARTESIAN_POINT('Origin',(-5.,1.2,17.4));
#22354=CARTESIAN_POINT('',(-5.,1.2,16.6));
#22355=CARTESIAN_POINT('',(-5.,1.2,17.4));
#22356=CARTESIAN_POINT('',(5.,1.2,16.6));
#22357=CARTESIAN_POINT('Origin',(-5.,0.8,17.4));
#22358=CARTESIAN_POINT('',(-5.,1.2,16.6));
#22359=CARTESIAN_POINT('Origin',(0.,1.,16.6));
#22360=CARTESIAN_POINT('Origin',(5.,1.6,17.4));
#22361=CARTESIAN_POINT('',(5.,1.6,16.6));
#22362=CARTESIAN_POINT('',(5.,1.6,17.4));
#22363=CARTESIAN_POINT('',(-5.,1.6,16.6));
#22364=CARTESIAN_POINT('',(-5.,1.6,16.6));
#22365=CARTESIAN_POINT('',(-5.,1.6,17.4));
#22366=CARTESIAN_POINT('Origin',(5.,2.,17.4));
#22367=CARTESIAN_POINT('',(5.,2.,16.6));
#22368=CARTESIAN_POINT('',(5.,2.,17.4));
#22369=CARTESIAN_POINT('',(5.,1.6,16.6));
#22370=CARTESIAN_POINT('Origin',(-5.,2.,17.4));
#22371=CARTESIAN_POINT('',(-5.,2.,16.6));
#22372=CARTESIAN_POINT('',(-5.,2.,17.4));
#22373=CARTESIAN_POINT('',(5.,2.,16.6));
#22374=CARTESIAN_POINT('Origin',(-5.,1.6,17.4));
#22375=CARTESIAN_POINT('',(-5.,2.,16.6));
#22376=CARTESIAN_POINT('Origin',(0.,1.8,16.6));
#22377=CARTESIAN_POINT('Origin',(5.,2.4,17.4));
#22378=CARTESIAN_POINT('',(5.,2.4,16.6));
#22379=CARTESIAN_POINT('',(5.,2.4,17.4));
#22380=CARTESIAN_POINT('',(-5.,2.4,16.6));
#22381=CARTESIAN_POINT('',(-5.,2.4,16.6));
#22382=CARTESIAN_POINT('',(-5.,2.4,17.4));
#22383=CARTESIAN_POINT('Origin',(5.,2.8,17.4));
#22384=CARTESIAN_POINT('',(5.,2.8,16.6));
#22385=CARTESIAN_POINT('',(5.,2.8,17.4));
#22386=CARTESIAN_POINT('',(5.,2.4,16.6));
#22387=CARTESIAN_POINT('Origin',(-5.,2.8,17.4));
#22388=CARTESIAN_POINT('',(-5.,2.8,16.6));
#22389=CARTESIAN_POINT('',(-5.,2.8,17.4));
#22390=CARTESIAN_POINT('',(5.,2.8,16.6));
#22391=CARTESIAN_POINT('Origin',(-5.,2.4,17.4));
#22392=CARTESIAN_POINT('',(-5.,2.8,16.6));
#22393=CARTESIAN_POINT('Origin',(0.,2.6,16.6));
#22394=CARTESIAN_POINT('Origin',(5.,-1.2,17.4));
#22395=CARTESIAN_POINT('',(5.,-1.2,16.6));
#22396=CARTESIAN_POINT('',(5.,-1.2,17.4));
#22397=CARTESIAN_POINT('',(-5.,-1.2,16.6));
#22398=CARTESIAN_POINT('',(-5.,-1.2,16.6));
#22399=CARTESIAN_POINT('',(-5.,-1.2,17.4));
#22400=CARTESIAN_POINT('Origin',(5.,-0.8,17.4));
#22401=CARTESIAN_POINT('',(5.,-0.8,16.6));
#22402=CARTESIAN_POINT('',(5.,-0.8,17.4));
#22403=CARTESIAN_POINT('',(5.,-1.2,16.6));
#22404=CARTESIAN_POINT('Origin',(-5.,-0.8,17.4));
#22405=CARTESIAN_POINT('',(-5.,-0.8,16.6));
#22406=CARTESIAN_POINT('',(-5.,-0.8,17.4));
#22407=CARTESIAN_POINT('',(5.,-0.8,16.6));
#22408=CARTESIAN_POINT('Origin',(-5.,-1.2,17.4));
#22409=CARTESIAN_POINT('',(-5.,-0.8,16.6));
#22410=CARTESIAN_POINT('Origin',(0.,-1.,16.6));
#22411=CARTESIAN_POINT('Origin',(5.,-2.8,17.4));
#22412=CARTESIAN_POINT('',(5.,-2.8,16.6));
#22413=CARTESIAN_POINT('',(5.,-2.8,17.4));
#22414=CARTESIAN_POINT('',(-5.,-2.8,16.6));
#22415=CARTESIAN_POINT('',(-5.,-2.8,16.6));
#22416=CARTESIAN_POINT('',(-5.,-2.8,17.4));
#22417=CARTESIAN_POINT('Origin',(5.,-2.4,17.4));
#22418=CARTESIAN_POINT('',(5.,-2.4,16.6));
#22419=CARTESIAN_POINT('',(5.,-2.4,17.4));
#22420=CARTESIAN_POINT('',(5.,-2.8,16.6));
#22421=CARTESIAN_POINT('Origin',(-5.,-2.4,17.4));
#22422=CARTESIAN_POINT('',(-5.,-2.4,16.6));
#22423=CARTESIAN_POINT('',(-5.,-2.4,17.4));
#22424=CARTESIAN_POINT('',(5.,-2.4,16.6));
#22425=CARTESIAN_POINT('Origin',(-5.,-2.8,17.4));
#22426=CARTESIAN_POINT('',(-5.,-2.4,16.6));
#22427=CARTESIAN_POINT('Origin',(0.,-2.6,16.6));
#22428=CARTESIAN_POINT('Origin',(6.5575,0.,13.5));
#22429=CARTESIAN_POINT('',(5.915,-3.18408167778312E-16,10.9));
#22430=CARTESIAN_POINT('',(6.5575,-3.18408167778312E-16,10.9));
#22431=CARTESIAN_POINT('Origin',(5.915,0.,13.5));
#22432=CARTESIAN_POINT('Origin',(5.915,0.,16.25));
#22433=CARTESIAN_POINT('',(5.915,-3.36777869765522E-16,10.75));
#22434=CARTESIAN_POINT('Origin',(5.915,0.,13.5));
#22435=CARTESIAN_POINT('Origin',(5.8075,0.,13.5));
#22436=CARTESIAN_POINT('',(5.7,-3.36777869765522E-16,10.75));
#22437=CARTESIAN_POINT('',(5.8075,-3.36777869765522E-16,10.75));
#22438=CARTESIAN_POINT('Origin',(5.7,0.,13.5));
#22439=CARTESIAN_POINT('Origin',(5.7,0.,16.1));
#22440=CARTESIAN_POINT('',(5.7,-3.18408167778312E-16,10.9));
#22441=CARTESIAN_POINT('Origin',(5.7,0.,13.5));
#22442=CARTESIAN_POINT('Origin',(5.05,0.,13.5));
#22443=CARTESIAN_POINT('',(4.4,-3.18408167778312E-16,10.9));
#22444=CARTESIAN_POINT('',(5.05,-3.18408167778312E-16,10.9));
#22445=CARTESIAN_POINT('Origin',(4.4,0.,13.5));
#22446=CARTESIAN_POINT('Origin',(4.4,0.,15.8));
#22447=CARTESIAN_POINT('',(4.4,-2.81668763803891E-16,11.2));
#22448=CARTESIAN_POINT('Origin',(4.4,0.,13.5));
#22449=CARTESIAN_POINT('Origin',(0.,0.,13.5));
#22450=CARTESIAN_POINT('',(3.47706773014274,-1.40834381901946E-16,11.2));
#22451=CARTESIAN_POINT('',(0.,-2.81668763803891E-16,11.2));
#22452=CARTESIAN_POINT('',(1.66533453693773E-16,-2.0712315177208,12.5));
#22453=CARTESIAN_POINT('Ctrl Pts',(0.,-2.0712315177208,12.5));
#22454=CARTESIAN_POINT('Ctrl Pts',(0.29627842792801,-2.0712315177208,12.5));
#22455=CARTESIAN_POINT('Ctrl Pts',(0.601922961286425,-2.05958767676481,
12.4745443794946));
#22456=CARTESIAN_POINT('Ctrl Pts',(1.20334931546476,-2.00447274662769,12.3705976495442));
#22457=CARTESIAN_POINT('Ctrl Pts',(1.49912274563406,-1.96094879925114,12.292086027079));
#22458=CARTESIAN_POINT('Ctrl Pts',(2.05395568676163,-1.82468777995446,12.0946869078541));
#22459=CARTESIAN_POINT('Ctrl Pts',(2.31304412039431,-1.73185180887424,11.9758067799491));
#22460=CARTESIAN_POINT('Ctrl Pts',(2.77233292995656,-1.47332713087679,11.7246738665425));
#22461=CARTESIAN_POINT('Ctrl Pts',(2.97292007577089,-1.30853389661232,11.5922075947285));
#22462=CARTESIAN_POINT('Ctrl Pts',(3.18569785359246,-1.01845799849145,11.4362114294288));
#22463=CARTESIAN_POINT('Ctrl Pts',(3.23470613609049,-0.939780894043197,
11.398772551631));
#22464=CARTESIAN_POINT('Ctrl Pts',(3.32099876549632,-0.770171936350533,
11.3308572866818));
#22465=CARTESIAN_POINT('Ctrl Pts',(3.35829264222579,-0.679232393641301,
11.300412215585));
#22466=CARTESIAN_POINT('Ctrl Pts',(3.41804439766507,-0.490271405037467,
11.2507383977881));
#22467=CARTESIAN_POINT('Ctrl Pts',(3.44056498067965,-0.392091297884813,
11.2314874762236));
#22468=CARTESIAN_POINT('Ctrl Pts',(3.47007525605945,-0.19487349905874,11.2061148726341));
#22469=CARTESIAN_POINT('Ctrl Pts',(3.47706773014274,-0.0958353476442229,
11.2));
#22470=CARTESIAN_POINT('Ctrl Pts',(3.47706773014274,-2.77555756156289E-17,
11.2));
#22471=CARTESIAN_POINT('',(-3.47706773014274,-1.40834381901946E-16,11.2));
#22472=CARTESIAN_POINT('Ctrl Pts',(-3.47706773014274,0.,11.2));
#22473=CARTESIAN_POINT('Ctrl Pts',(-3.47706773014274,-0.0958353476442226,
11.2));
#22474=CARTESIAN_POINT('Ctrl Pts',(-3.47007525605945,-0.194873499058739,
11.2061148726341));
#22475=CARTESIAN_POINT('Ctrl Pts',(-3.44056498067966,-0.392091297884812,
11.2314874762236));
#22476=CARTESIAN_POINT('Ctrl Pts',(-3.41804439766507,-0.490271405037466,
11.2507383977881));
#22477=CARTESIAN_POINT('Ctrl Pts',(-3.35829264222578,-0.679232393641301,
11.300412215585));
#22478=CARTESIAN_POINT('Ctrl Pts',(-3.32099876549632,-0.770171936350533,
11.3308572866818));
#22479=CARTESIAN_POINT('Ctrl Pts',(-3.23470613609049,-0.939780894043197,
11.398772551631));
#22480=CARTESIAN_POINT('Ctrl Pts',(-3.18569785359246,-1.01845799849145,
11.4362114294288));
#22481=CARTESIAN_POINT('Ctrl Pts',(-2.97292007577089,-1.30853389661232,
11.5922075947285));
#22482=CARTESIAN_POINT('Ctrl Pts',(-2.77233292995656,-1.47332713087679,
11.7246738665425));
#22483=CARTESIAN_POINT('Ctrl Pts',(-2.31304412039431,-1.73185180887424,
11.9758067799491));
#22484=CARTESIAN_POINT('Ctrl Pts',(-2.05395568676163,-1.82468777995446,
12.0946869078541));
#22485=CARTESIAN_POINT('Ctrl Pts',(-1.49912274563406,-1.96094879925114,
12.292086027079));
#22486=CARTESIAN_POINT('Ctrl Pts',(-1.20334931546476,-2.00447274662769,
12.3705976495442));
#22487=CARTESIAN_POINT('Ctrl Pts',(-0.601922961286425,-2.05958767676481,
12.4745443794946));
#22488=CARTESIAN_POINT('Ctrl Pts',(-0.29627842792801,-2.0712315177208,12.5));
#22489=CARTESIAN_POINT('Ctrl Pts',(0.,-2.0712315177208,12.5));
#22490=CARTESIAN_POINT('',(-4.4,-2.81668763803891E-16,11.2));
#22491=CARTESIAN_POINT('',(0.,-2.81668763803891E-16,11.2));
#22492=CARTESIAN_POINT('Origin',(-4.4,0.,13.5));
#22493=CARTESIAN_POINT('Ctrl Pts',(3.47706773014274,-5.55111512312578E-17,
11.2));
#22494=CARTESIAN_POINT('Ctrl Pts',(3.47706773014274,0.0958353476442228,
11.2));
#22495=CARTESIAN_POINT('Ctrl Pts',(3.47007525605945,0.194873499058739,11.2061148726341));
#22496=CARTESIAN_POINT('Ctrl Pts',(3.44056498067965,0.392091297884812,11.2314874762236));
#22497=CARTESIAN_POINT('Ctrl Pts',(3.41804439766507,0.490271405037467,11.2507383977881));
#22498=CARTESIAN_POINT('Ctrl Pts',(3.35829264222579,0.679232393641301,11.300412215585));
#22499=CARTESIAN_POINT('Ctrl Pts',(3.32099876549632,0.770171936350533,11.3308572866818));
#22500=CARTESIAN_POINT('Ctrl Pts',(3.23470613609049,0.939780894043197,11.398772551631));
#22501=CARTESIAN_POINT('Ctrl Pts',(3.18569785359246,1.01845799849145,11.4362114294288));
#22502=CARTESIAN_POINT('Ctrl Pts',(2.97292007577089,1.30853389661232,11.5922075947285));
#22503=CARTESIAN_POINT('Ctrl Pts',(2.77233292995656,1.47332713087679,11.7246738665425));
#22504=CARTESIAN_POINT('Ctrl Pts',(2.31304412039431,1.73185180887424,11.9758067799491));
#22505=CARTESIAN_POINT('Ctrl Pts',(2.05395568676163,1.82468777995446,12.0946869078541));
#22506=CARTESIAN_POINT('Ctrl Pts',(1.49912274563406,1.96094879925114,12.292086027079));
#22507=CARTESIAN_POINT('Ctrl Pts',(1.20334931546476,2.00447274662769,12.3705976495442));
#22508=CARTESIAN_POINT('Ctrl Pts',(0.601922961286424,2.05958767676481,12.4745443794946));
#22509=CARTESIAN_POINT('Ctrl Pts',(0.29627842792801,2.0712315177208,12.5));
#22510=CARTESIAN_POINT('Ctrl Pts',(0.,2.0712315177208,12.5));
#22511=CARTESIAN_POINT('Ctrl Pts',(-0.29627842792801,2.0712315177208,12.5));
#22512=CARTESIAN_POINT('Ctrl Pts',(-0.601922961286424,2.05958767676481,
12.4745443794946));
#22513=CARTESIAN_POINT('Ctrl Pts',(-1.20334931546475,2.00447274662769,12.3705976495442));
#22514=CARTESIAN_POINT('Ctrl Pts',(-1.49912274563406,1.96094879925114,12.292086027079));
#22515=CARTESIAN_POINT('Ctrl Pts',(-2.05395568676163,1.82468777995446,12.0946869078541));
#22516=CARTESIAN_POINT('Ctrl Pts',(-2.31304412039431,1.73185180887424,11.9758067799491));
#22517=CARTESIAN_POINT('Ctrl Pts',(-2.77233292995656,1.47332713087679,11.7246738665425));
#22518=CARTESIAN_POINT('Ctrl Pts',(-2.97292007577089,1.30853389661232,11.5922075947285));
#22519=CARTESIAN_POINT('Ctrl Pts',(-3.18569785359246,1.01845799849145,11.4362114294288));
#22520=CARTESIAN_POINT('Ctrl Pts',(-3.23470613609049,0.939780894043197,
11.398772551631));
#22521=CARTESIAN_POINT('Ctrl Pts',(-3.32099876549632,0.770171936350533,
11.3308572866818));
#22522=CARTESIAN_POINT('Ctrl Pts',(-3.35829264222578,0.679232393641301,
11.300412215585));
#22523=CARTESIAN_POINT('Ctrl Pts',(-3.41804439766507,0.490271405037466,
11.2507383977881));
#22524=CARTESIAN_POINT('Ctrl Pts',(-3.44056498067966,0.392091297884812,
11.2314874762236));
#22525=CARTESIAN_POINT('Ctrl Pts',(-3.47007525605945,0.194873499058739,
11.2061148726341));
#22526=CARTESIAN_POINT('Ctrl Pts',(-3.47706773014274,0.0958353476442226,
11.2));
#22527=CARTESIAN_POINT('Ctrl Pts',(-3.47706773014274,2.77555756156289E-17,
11.2));
#22528=CARTESIAN_POINT('Origin',(-4.4,0.,16.1));
#22529=CARTESIAN_POINT('',(-4.4,-3.18408167778312E-16,10.9));
#22530=CARTESIAN_POINT('Origin',(-4.4,0.,13.5));
#22531=CARTESIAN_POINT('Origin',(-5.05,0.,13.5));
#22532=CARTESIAN_POINT('',(-5.7,-3.18408167778312E-16,10.9));
#22533=CARTESIAN_POINT('',(-5.05,-3.18408167778312E-16,10.9));
#22534=CARTESIAN_POINT('Origin',(-5.7,0.,13.5));
#22535=CARTESIAN_POINT('Origin',(-5.7,0.,16.25));
#22536=CARTESIAN_POINT('',(-5.7,-3.36777869765522E-16,10.75));
#22537=CARTESIAN_POINT('Origin',(-5.7,0.,13.5));
#22538=CARTESIAN_POINT('Origin',(-5.8075,0.,13.5));
#22539=CARTESIAN_POINT('',(-5.915,-3.36777869765522E-16,10.75));
#22540=CARTESIAN_POINT('',(-5.8075,-3.36777869765522E-16,10.75));
#22541=CARTESIAN_POINT('Origin',(-5.915,0.,13.5));
#22542=CARTESIAN_POINT('Origin',(-5.915,0.,16.1));
#22543=CARTESIAN_POINT('',(-5.915,-3.18408167778312E-16,10.9));
#22544=CARTESIAN_POINT('Origin',(-5.915,0.,13.5));
#22545=CARTESIAN_POINT('Origin',(-6.5575,0.,13.5));
#22546=CARTESIAN_POINT('',(-6.5575,-3.18408167778312E-16,10.9));
#22547=CARTESIAN_POINT('Origin',(0.,-1.25,7.2));
#22548=CARTESIAN_POINT('',(-6.49062803548097E-16,2.2,1.9));
#22549=CARTESIAN_POINT('',(-6.49062803548097E-16,-1.25,1.9));
#22550=CARTESIAN_POINT('Origin',(0.,2.2,7.2));
#22551=CARTESIAN_POINT('Origin',(0.,2.2,10.95));
#22552=CARTESIAN_POINT('',(-4.59242549680257E-16,2.2,3.45));
#22553=CARTESIAN_POINT('Origin',(0.,2.2,7.2));
#22554=CARTESIAN_POINT('Origin',(0.,3.5,7.2));
#22555=CARTESIAN_POINT('',(-4.59242549680257E-16,4.8,3.45));
#22556=CARTESIAN_POINT('',(-4.59242549680257E-16,3.5,3.45));
#22557=CARTESIAN_POINT('Origin',(0.,4.8,7.2));
#22558=CARTESIAN_POINT('Origin',(0.,4.8,10.3));
#22559=CARTESIAN_POINT('',(-3.7964050773568E-16,4.8,4.1));
#22560=CARTESIAN_POINT('Origin',(0.,4.8,7.2));
#22561=CARTESIAN_POINT('Origin',(0.,5.175,7.2));
#22562=CARTESIAN_POINT('',(-3.7964050773568E-16,5.55,4.1));
#22563=CARTESIAN_POINT('',(-3.79640507735679E-16,5.175,4.1));
#22564=CARTESIAN_POINT('Origin',(0.,5.55,7.2));
#22565=CARTESIAN_POINT('Origin',(0.,5.605,7.2));
#22566=CARTESIAN_POINT('',(-3.8637606513099E-16,5.605,4.045));
#22567=CARTESIAN_POINT('Origin',(0.,4.6,7.2));
#22568=CARTESIAN_POINT('Origin',(6.6,0.,0.6));
#22569=CARTESIAN_POINT('Origin',(-6.6,0.,0.6));
#86391=UNCERTAINTY_MEASURE_WITH_UNIT(LENGTH_MEASURE(0.001),#86430,
'DISTANCE_ACCURACY_VALUE',
'Maximum model space distance between geometric entities at asserted c
onnectivities');
#86409=UNCERTAINTY_MEASURE_WITH_UNIT(LENGTH_MEASURE(0.001),#86430,
'DISTANCE_ACCURACY_VALUE',
'Maximum model space distance between geometric entities at asserted c
onnectivities');
#86411=(
GEOMETRIC_REPRESENTATION_CONTEXT(3)
GLOBAL_UNCERTAINTY_ASSIGNED_CONTEXT((#86391))
GLOBAL_UNIT_ASSIGNED_CONTEXT((#86430,#86432,#86433))
REPRESENTATION_CONTEXT('','3D')
);
#86429=(
GEOMETRIC_REPRESENTATION_CONTEXT(3)
GLOBAL_UNCERTAINTY_ASSIGNED_CONTEXT((#86409))
GLOBAL_UNIT_ASSIGNED_CONTEXT((#86430,#86432,#86433))
REPRESENTATION_CONTEXT('','3D')
);
#86430=(
LENGTH_UNIT()
NAMED_UNIT(*)
SI_UNIT(.CENTI.,.METRE.)
);
#86432=(
NAMED_UNIT(*)
PLANE_ANGLE_UNIT()
SI_UNIT($,.RADIAN.)
);
#86433=(
NAMED_UNIT(*)
SI_UNIT($,.STERADIAN.)
SOLID_ANGLE_UNIT()
);
#86435=SHAPE_DEFINITION_REPRESENTATION(#86454,#86502);
#86454=PRODUCT_DEFINITION_SHAPE('',$,#86522);
#86502=SHAPE_REPRESENTATION('',(#15831),#86411);
#86520=PRODUCT_DEFINITION_CONTEXT('part definition',#86579,'design');
#86522=PRODUCT_DEFINITION('Housing','Housing',#86541,#86520);
#86541=PRODUCT_DEFINITION_FORMATION('',$,#86582);
#86579=APPLICATION_CONTEXT(
'Core Data for Automotive Mechanical Design Process');
#86580=PRODUCT_CONTEXT('part definition',#86579,'mechanical');
#86582=PRODUCT('Housing','Housing',$,(#86580));
#86601=PRESENTATION_STYLE_ASSIGNMENT((#86619));
#86619=SURFACE_STYLE_USAGE(.BOTH.,#86637);
#86637=SURFACE_SIDE_STYLE('',(#86655));
#86655=SURFACE_STYLE_FILL_AREA(#86673);
#86673=FILL_AREA_STYLE('Opaque(192,195,199)',(#86691));
#86691=FILL_AREA_STYLE_COLOUR('Opaque(192,195,199)',#86709);
#86709=COLOUR_RGB('Opaque(192,195,199)', 0.09019608, 0.27058824, 0.51372549);
ENDSEC;
END-ISO-10303-21;
